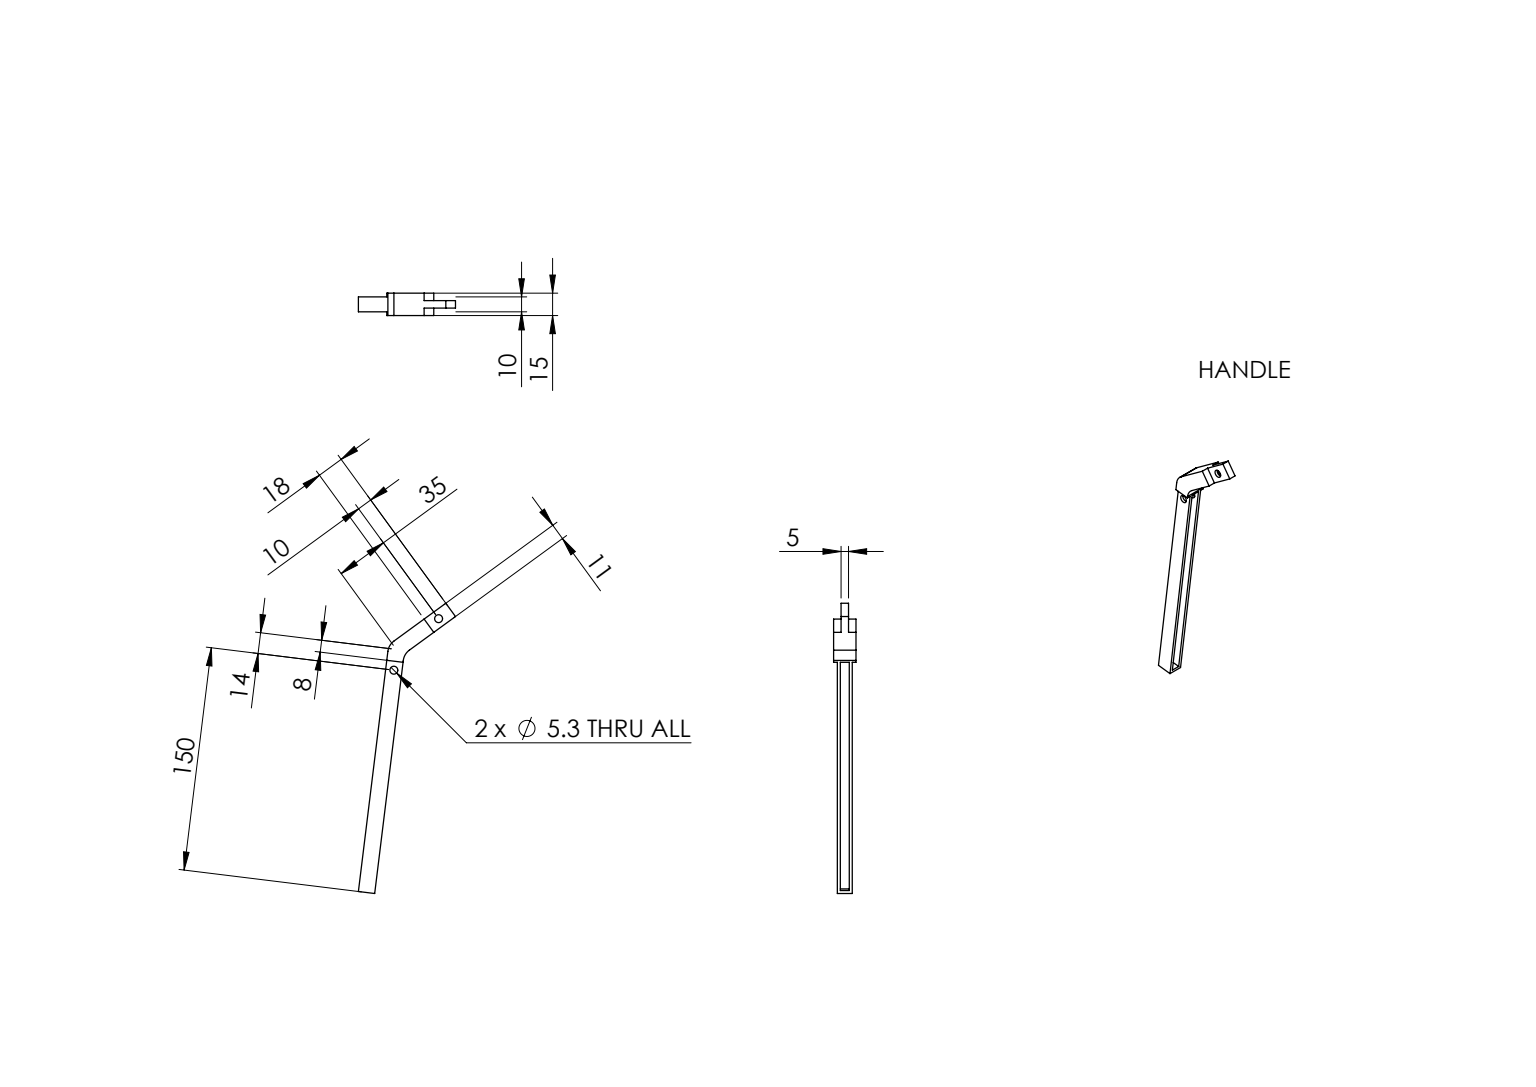
ISO-10303-21;
HEADER;
FILE_DESCRIPTION (('STEP AP214'),
    '1' );
FILE_NAME ('handle.step',
    '2026-10-31T03:36:27',
    ( '' ),
    ( '' ),
    'SwSTEP 2.0',
    'SolidWorks 2026',
    '' );
FILE_SCHEMA (( 'AUTOMOTIVE_DESIGN' ));
ENDSEC;

DATA;
#21=VERTEX_POINT ( 'NONE', #9252 ) ;
#62=EDGE_CURVE ( 'NONE', #31856, #6278, #12468, .T. ) ;
#113=VERTEX_POINT ( 'NONE', #15124 ) ;
#115=CARTESIAN_POINT ( 'NONE',  ( -98.52697526167152375, 63.53212182842481326, 3.000000000000000000 ) ) ;
#118=DIRECTION ( 'NONE',  ( -0.000000000000000000, 0.000000000000000000, 1.000000000000000000 ) ) ;
#138=PLANE ( 'NONE',  #16547 ) ;
#165=ADVANCED_FACE ( 'NONE', ( #28756 ), #138, .T. ) ;
#203=DIRECTION ( 'NONE',  ( 0.000000000000000000, 0.000000000000000000, -1.000000000000000000 ) ) ;
#232=ORIENTED_EDGE ( 'NONE', *, *, #9936, .F. ) ;
#254=ORIENTED_EDGE ( 'NONE', *, *, #1063, .F. ) ;
#301=LINE ( 'NONE', #23435, #5184 ) ;
#362=CYLINDRICAL_SURFACE ( 'NONE', #12150, 2.649999999999999467 ) ;
#375=FACE_OUTER_BOUND ( 'NONE', #36390, .T. ) ;
#384=FACE_BOUND ( 'NONE', #21248, .T. ) ;
#442=DIRECTION ( 'NONE',  ( 0.1219804832088915436, 0.9925324990730154395, 0.000000000000000000 ) ) ;
#456=VERTEX_POINT ( 'NONE', #12456 ) ;
#477=LINE ( 'NONE', #26256, #35797 ) ;
#513=DIRECTION ( 'NONE',  ( -0.8083506638593008775, -0.5887012860850803220, 0.000000000000000000 ) ) ;
#553=DIRECTION ( 'NONE',  ( 1.000000000000000000, 0.000000000000000000, 0.000000000000000000 ) ) ;
#622=EDGE_LOOP ( 'NONE', ( #9730, #27726, #18131, #5252 ) ) ;
#651=CARTESIAN_POINT ( 'NONE',  ( -70.80918835584510873, 215.2843023367891249, 3.000000000000000000 ) ) ;
#676=EDGE_CURVE ( 'NONE', #21562, #5473, #30076, .T. ) ;
#701=DIRECTION ( 'NONE',  ( 0.5887012860850814322, -0.8083506638592999893, 0.000000000000000000 ) ) ;
#743=DIRECTION ( 'NONE',  ( -0.000000000000000000, -0.000000000000000000, -1.000000000000000000 ) ) ;
#745=CARTESIAN_POINT ( 'NONE',  ( -44.35000000000001563, 244.5000000000000000, 5.000000000000000000 ) ) ;
#758=AXIS2_PLACEMENT_3D ( 'NONE', #36466, #33265, #18505 ) ;
#788=LINE ( 'NONE', #10083, #33967 ) ;
#790=EDGE_CURVE ( 'NONE', #30802, #1071, #21746, .T. ) ;
#796=LINE ( 'NONE', #12366, #13356 ) ;
#852=PLANE ( 'NONE',  #25668 ) ;
#858=AXIS2_PLACEMENT_3D ( 'NONE', #37408, #25218, #21126 ) ;
#894=EDGE_CURVE ( 'NONE', #12557, #11771, #34221, .T. ) ;
#916=AXIS2_PLACEMENT_3D ( 'NONE', #4687, #25159, #10753 ) ;
#946=CARTESIAN_POINT ( 'NONE',  ( -95.81998461310567450, 11.77610610744882358, 3.000000000000000000 ) ) ;
#1022=EDGE_CURVE ( 'NONE', #18726, #12845, #31747, .T. ) ;
#1057=LINE ( 'NONE', #12631, #35525 ) ;
#1063=EDGE_CURVE ( 'NONE', #6180, #9049, #14403, .T. ) ;
#1065=APPLICATION_CONTEXT ( 'automotive_design' ) ;
#1071=VERTEX_POINT ( 'NONE', #25874 ) ;
#1075=CARTESIAN_POINT ( 'NONE',  ( -76.95115755716804529, 229.4913094451872553, -7.500000000000000000 ) ) ;
#1204=AXIS2_PLACEMENT_3D ( 'NONE', #34736, #8411, #23189 ) ;
#1274=ORIENTED_EDGE ( 'NONE', *, *, #16176, .T. ) ;
#1330=ORIENTED_EDGE ( 'NONE', *, *, #23016, .T. ) ;
#1365=CARTESIAN_POINT ( 'NONE',  ( -89.83814373643217266, 60.44923248139874516, 5.000000000000000000 ) ) ;
#1475=VERTEX_POINT ( 'NONE', #13339 ) ;
#1483=VECTOR ( 'NONE', #7906, 1000.000000000000000 ) ;
#1499=LINE ( 'NONE', #745, #33419 ) ;
#1501=CARTESIAN_POINT ( 'NONE',  ( -60.72871937935236986, 215.3268752544371978, 5.000000000000000000 ) ) ;
#1550=DIRECTION ( 'NONE',  ( -0.9925324990730152175, 0.1219804832088933616, 0.000000000000000000 ) ) ;
#1568=ORIENTED_EDGE ( 'NONE', *, *, #4516, .F. ) ;
#1589=EDGE_CURVE ( 'NONE', #25013, #11771, #16193, .T. ) ;
#1594=DIRECTION ( 'NONE',  ( -1.558072081575740353E-16, -1.134704379232807653E-16, -1.000000000000000000 ) ) ;
#1616=DIRECTION ( 'NONE',  ( -0.000000000000000000, -0.000000000000000000, -1.000000000000000000 ) ) ;
#1652=FACE_OUTER_BOUND ( 'NONE', #9339, .T. ) ;
#1664=ORIENTED_EDGE ( 'NONE', *, *, #36317, .F. ) ;
#1688=LINE ( 'NONE', #24815, #8796 ) ;
#1716=CARTESIAN_POINT ( 'NONE',  ( -79.65000000000000568, 210.0000000000000000, 5.000000000000000888 ) ) ;
#1759=EDGE_CURVE ( 'NONE', #19165, #27793, #2654, .T. ) ;
#1782=DIRECTION ( 'NONE',  ( 1.000000000000000000, 0.000000000000000000, 0.000000000000000000 ) ) ;
#1788=ORIENTED_EDGE ( 'NONE', *, *, #3607, .F. ) ;
#1826=VECTOR ( 'NONE', #29654, 1000.000000000000114 ) ;
#1846=DIRECTION ( 'NONE',  ( -0.5887012860850813212, 0.8083506638592999893, 0.000000000000000000 ) ) ;
#1872=CARTESIAN_POINT ( 'NONE',  ( -74.35000000000002274, 210.0000000000000000, 3.000000000000000000 ) ) ;
#1885=DIRECTION ( 'NONE',  ( -0.000000000000000000, -0.000000000000000000, 1.000000000000000000 ) ) ;
#1893=DIRECTION ( 'NONE',  ( 1.000000000000000000, 0.000000000000000000, 0.000000000000000000 ) ) ;
#1965=CYLINDRICAL_SURFACE ( 'NONE', #29291, 2.649999999999992806 ) ;
#1966=CARTESIAN_POINT ( 'NONE',  ( -44.35000000000001563, 244.5000000000000000, -2.499999999999998224 ) ) ;
#1984=VERTEX_POINT ( 'NONE', #17641 ) ;
#2027=CARTESIAN_POINT ( 'NONE',  ( -74.35000000000002274, 210.0000000000000000, 5.000000000000000000 ) ) ;
#2063=ADVANCED_FACE ( 'NONE', ( #24072 ), #6442, .T. ) ;
#2067=ORIENTED_EDGE ( 'NONE', *, *, #6952, .T. ) ;
#2076=DIRECTION ( 'NONE',  ( 1.000000000000000000, 0.000000000000000000, 0.000000000000000000 ) ) ;
#2157=ORIENTED_EDGE ( 'NONE', *, *, #11690, .F. ) ;
#2200=PLANE ( 'NONE',  #31590 ) ;
#2202=DIRECTION ( 'NONE',  ( -1.000000000000000000, 0.000000000000000000, 0.000000000000000000 ) ) ;
#2225=ADVANCED_FACE ( 'NONE', ( #12877 ), #29745, .F. ) ;
#2246=DIRECTION ( 'NONE',  ( 0.000000000000000000, 0.000000000000000000, -1.000000000000000000 ) ) ;
#2286=DIRECTION ( 'NONE',  ( 0.000000000000000000, 0.000000000000000000, -1.000000000000000000 ) ) ;
#2390=CARTESIAN_POINT ( 'NONE',  ( -77.00000000000002842, 210.0000000000000000, -3.000000000000000000 ) ) ;
#2409=CARTESIAN_POINT ( 'NONE',  ( -82.45892874490161262, 210.6708926576488921, 5.000000000000000000 ) ) ;
#2412=EDGE_CURVE ( 'NONE', #21814, #23956, #15632, .T. ) ;
#2424=DIRECTION ( 'NONE',  ( -0.5887012860850800999, 0.8083506638593009885, 0.000000000000000000 ) ) ;
#2432=FACE_OUTER_BOUND ( 'NONE', #27389, .T. ) ;
#2469=CARTESIAN_POINT ( 'NONE',  ( -56.70466238434235606, 244.2363183625454894, -7.500000000000000000 ) ) ;
#2501=DIRECTION ( 'NONE',  ( 1.000000000000000000, 0.000000000000000000, 0.000000000000000000 ) ) ;
#2524=VECTOR ( 'NONE', #12034, 1000.000000000000000 ) ;
#2544=ORIENTED_EDGE ( 'NONE', *, *, #13634, .T. ) ;
#2564=ORIENTED_EDGE ( 'NONE', *, *, #9364, .F. ) ;
#2574=DIRECTION ( 'NONE',  ( -0.5887012860850800999, 0.8083506638593009885, -0.000000000000000000 ) ) ;
#2638=SHAPE_REPRESENTATION ( 'handle', ( #17215 ), #15973 ) ;
#2654=LINE ( 'NONE', #3216, #27316 ) ;
#2669=VECTOR ( 'NONE', #5948, 1000.000000000000000 ) ;
#2747=DIRECTION ( 'NONE',  ( -0.1219804832088935975, -0.9925324990730152175, 0.000000000000000000 ) ) ;
#2750=VECTOR ( 'NONE', #5758, 1000.000000000000000 ) ;
#2820=EDGE_LOOP ( 'NONE', ( #232, #22651, #21479, #3234 ) ) ;
#2857=ORIENTED_EDGE ( 'NONE', *, *, #34192, .F. ) ;
#2926=EDGE_CURVE ( 'NONE', #4785, #26168, #26714, .T. ) ;
#2932=DIRECTION ( 'NONE',  ( -1.000000000000000000, 0.000000000000000000, 1.636531581110199847E-16 ) ) ;
#2967=DIRECTION ( 'NONE',  ( -0.5887012860850802110, 0.8083506638593009885, 0.000000000000000000 ) ) ;
#2988=DIRECTION ( 'NONE',  ( -0.5887012860850802110, 0.8083506638593008775, 2.465190328815661618E-32 ) ) ;
#3046=ORIENTED_EDGE ( 'NONE', *, *, #24454, .T. ) ;
#3079=DIRECTION ( 'NONE',  ( -1.000000000000000000, 2.775557561562892929E-15, 0.000000000000000000 ) ) ;
#3082=PLANE ( 'NONE',  #1204 ) ;
#3099=ORIENTED_EDGE ( 'NONE', *, *, #7158, .T. ) ;
#3104=EDGE_CURVE ( 'NONE', #9049, #11398, #1499, .T. ) ;
#3106=DIRECTION ( 'NONE',  ( 0.1219804832088915436, 0.9925324990730154395, 0.000000000000000000 ) ) ;
#3138=AXIS2_PLACEMENT_3D ( 'NONE', #4717, #16110, #19522 ) ;
#3147=VERTEX_POINT ( 'NONE', #13825 ) ;
#3216=CARTESIAN_POINT ( 'NONE',  ( -74.35000000000002274, 210.0000000000000000, 5.000000000000000000 ) ) ;
#3234=ORIENTED_EDGE ( 'NONE', *, *, #32163, .F. ) ;
#3331=ORIENTED_EDGE ( 'NONE', *, *, #24454, .F. ) ;
#3343=ADVANCED_FACE ( 'NONE', ( #2432 ), #22730, .T. ) ;
#3349=EDGE_CURVE ( 'NONE', #18726, #12557, #28030, .T. ) ;
#3423=ORIENTED_EDGE ( 'NONE', *, *, #25829, .F. ) ;
#3598=CARTESIAN_POINT ( 'NONE',  ( -70.80918835584510873, 215.2843023367891249, 7.500000000000000000 ) ) ;
#3607=EDGE_CURVE ( 'NONE', #28581, #26637, #20070, .T. ) ;
#3645=LINE ( 'NONE', #6873, #19995 ) ;
#3688=CIRCLE ( 'NONE', #5491, 2.649999999999992806 ) ;
#3707=ORIENTED_EDGE ( 'NONE', *, *, #21878, .T. ) ;
#3805=AXIS2_PLACEMENT_3D ( 'NONE', #2409, #25905, #5616 ) ;
#3827=VERTEX_POINT ( 'NONE', #6976 ) ;
#3831=LINE ( 'NONE', #18826, #25418 ) ;
#3848=ORIENTED_EDGE ( 'NONE', *, *, #5518, .T. ) ;
#3850=ORIENTED_EDGE ( 'NONE', *, *, #8314, .T. ) ;
#3879=DIRECTION ( 'NONE',  ( -0.9925324990730152175, 0.1219804832088933616, 0.000000000000000000 ) ) ;
#3926=EDGE_CURVE ( 'NONE', #13097, #35545, #6587, .T. ) ;
#3932=DIRECTION ( 'NONE',  ( 0.9925324990730152175, -0.1219804832088933616, 0.000000000000000000 ) ) ;
#3950=AXIS2_PLACEMENT_3D ( 'NONE', #1501, #4347, #32971 ) ;
#3967=DIRECTION ( 'NONE',  ( -0.1219804832088933616, -0.9925324990730152175, 0.000000000000000000 ) ) ;
#3995=EDGE_LOOP ( 'NONE', ( #16459, #23432, #36012, #20738 ) ) ;
#3999=CIRCLE ( 'NONE', #28217, 2.649999999999999467 ) ;
#4055=ADVANCED_FACE ( 'NONE', ( #9806 ), #27055, .F. ) ;
#4063=VECTOR ( 'NONE', #21364, 1000.000000000000000 ) ;
#4074=ORIENTED_EDGE ( 'NONE', *, *, #23631, .F. ) ;
#4076=DIRECTION ( 'NONE',  ( -1.558072081575740353E-16, -1.134704379232807653E-16, -1.000000000000000000 ) ) ;
#4109=EDGE_LOOP ( 'NONE', ( #17978, #4758, #11450, #28178 ) ) ;
#4112=FACE_BOUND ( 'NONE', #26718, .T. ) ;
#4160=DIRECTION ( 'NONE',  ( -0.000000000000000000, -0.000000000000000000, 1.000000000000000000 ) ) ;
#4165=CARTESIAN_POINT ( 'NONE',  ( 25.01079625726091749, 203.5081962293401148, -5.000000000000000000 ) ) ;
#4229=CIRCLE ( 'NONE', #23608, 2.649999999999999467 ) ;
#4295=DIRECTION ( 'NONE',  ( 1.000000000000000000, 0.000000000000000000, 0.000000000000000000 ) ) ;
#4316=FACE_OUTER_BOUND ( 'NONE', #9865, .T. ) ;
#4344=DIRECTION ( 'NONE',  ( -0.9925324990730152175, 0.1219804832088933616, 0.000000000000000000 ) ) ;
#4347=DIRECTION ( 'NONE',  ( 0.000000000000000000, 0.000000000000000000, 1.000000000000000000 ) ) ;
#4367=ADVANCED_FACE ( 'NONE', ( #28170 ), #2200, .F. ) ;
#4393=PLANE ( 'NONE',  #29689 ) ;
#4397=CARTESIAN_POINT ( 'NONE',  ( -44.35000000000001563, 244.5000000000000000, 0.4999999999999995559 ) ) ;
#4410=ORIENTED_EDGE ( 'NONE', *, *, #6952, .F. ) ;
#4414=CIRCLE ( 'NONE', #34663, 2.649999999999999467 ) ;
#4423=CARTESIAN_POINT ( 'NONE',  ( -71.06414469631722852, 221.4078028065942476, -7.500000000000000888 ) ) ;
#4516=EDGE_CURVE ( 'NONE', #10660, #6278, #34966, .T. ) ;
#4546=CARTESIAN_POINT ( 'NONE',  ( -70.80918835584510873, 215.2843023367891249, -7.500000000000000000 ) ) ;
#4550=VERTEX_POINT ( 'NONE', #20205 ) ;
#4577=EDGE_CURVE ( 'NONE', #10335, #5564, #37064, .T. ) ;
#4625=LINE ( 'NONE', #9762, #14797 ) ;
#4643=DIRECTION ( 'NONE',  ( 0.000000000000000000, 0.000000000000000000, -1.000000000000000000 ) ) ;
#4651=DIRECTION ( 'NONE',  ( 0.000000000000000000, 0.000000000000000000, 1.000000000000000000 ) ) ;
#4661=ORIENTED_EDGE ( 'NONE', *, *, #25880, .F. ) ;
#4665=CARTESIAN_POINT ( 'NONE',  ( -70.80918835584510873, 215.2843023367891249, 7.500000000000000000 ) ) ;
#4681=VERTEX_POINT ( 'NONE', #22866 ) ;
#4687=CARTESIAN_POINT ( 'NONE',  ( -80.47386374675558329, 210.4269316912311183, 5.000000000000000000 ) ) ;
#4717=CARTESIAN_POINT ( 'NONE',  ( 38.04237167757703020, 114.1383727779938511, -2.499999999999996447 ) ) ;
#4722=VERTEX_POINT ( 'NONE', #29467 ) ;
#4736=ORIENTED_EDGE ( 'NONE', *, *, #8440, .F. ) ;
#4750=DIRECTION ( 'NONE',  ( -0.8083506638593009885, -0.5887012860850802110, 0.000000000000000000 ) ) ;
#4758=ORIENTED_EDGE ( 'NONE', *, *, #19169, .T. ) ;
#4785=VERTEX_POINT ( 'NONE', #651 ) ;
#4825=ORIENTED_EDGE ( 'NONE', *, *, #7158, .F. ) ;
#4865=DIRECTION ( 'NONE',  ( 1.000000000000000000, 0.000000000000000000, 0.000000000000000000 ) ) ;
#4942=EDGE_CURVE ( 'NONE', #14336, #33921, #9572, .T. ) ;
#5063=CIRCLE ( 'NONE', #33524, 9.999999999999994671 ) ;
#5102=CARTESIAN_POINT ( 'NONE',  ( -76.95115755716803108, 229.4913094451872553, 5.000000000000000000 ) ) ;
#5107=ORIENTED_EDGE ( 'NONE', *, *, #22482, .F. ) ;
#5134=ORIENTED_EDGE ( 'NONE', *, *, #8705, .F. ) ;
#5184=VECTOR ( 'NONE', #20982, 1000.000000000000000 ) ;
#5252=ORIENTED_EDGE ( 'NONE', *, *, #3926, .F. ) ;
#5262=EDGE_CURVE ( 'NONE', #21814, #456, #16018, .T. ) ;
#5314=FACE_OUTER_BOUND ( 'NONE', #26570, .T. ) ;
#5334=EDGE_LOOP ( 'NONE', ( #13000, #35007, #20837, #34063 ) ) ;
#5346=CARTESIAN_POINT ( 'NONE',  ( -47.00000000000000711, 244.5000000000000000, 5.000000000000000000 ) ) ;
#5348=CARTESIAN_POINT ( 'NONE',  ( -77.35272773637332477, 226.7246823105297153, -0.4999999999999908962 ) ) ;
#5426=EDGE_CURVE ( 'NONE', #1984, #18726, #26847, .T. ) ;
#5456=CARTESIAN_POINT ( 'NONE',  ( -50.22894823740646331, 235.3444610600932094, 7.500000000000000000 ) ) ;
#5473=VERTEX_POINT ( 'NONE', #34182 ) ;
#5491=AXIS2_PLACEMENT_3D ( 'NONE', #15956, #21462, #20892 ) ;
#5503=LINE ( 'NONE', #28625, #32722 ) ;
#5518=EDGE_CURVE ( 'NONE', #30233, #22653, #29035, .T. ) ;
#5524=CARTESIAN_POINT ( 'NONE',  ( -71.06414469631722852, 221.4078028065942476, 5.000000000000000000 ) ) ;
#5564=VERTEX_POINT ( 'NONE', #18257 ) ;
#5612=ORIENTED_EDGE ( 'NONE', *, *, #16982, .F. ) ;
#5616=DIRECTION ( 'NONE',  ( -0.1219804832088915297, -0.9925324990730154395, 0.000000000000000000 ) ) ;
#5758=DIRECTION ( 'NONE',  ( 0.000000000000000000, 0.000000000000000000, -1.000000000000000000 ) ) ;
#5889=ORIENTED_EDGE ( 'NONE', *, *, #4516, .T. ) ;
#5920=DIRECTION ( 'NONE',  ( -0.000000000000000000, -0.000000000000000000, -1.000000000000000000 ) ) ;
#5923=CARTESIAN_POINT ( 'NONE',  ( -44.35000000000001563, 244.5000000000000000, 2.500000000000000000 ) ) ;
#5948=DIRECTION ( 'NONE',  ( -0.000000000000000000, -0.000000000000000000, 1.000000000000000000 ) ) ;
#5989=ORIENTED_EDGE ( 'NONE', *, *, #7419, .T. ) ;
#6034=VERTEX_POINT ( 'NONE', #4397 ) ;
#6088=FACE_OUTER_BOUND ( 'NONE', #36886, .T. ) ;
#6146=VECTOR ( 'NONE', #20023, 1000.000000000000000 ) ;
#6168=ORIENTED_EDGE ( 'NONE', *, *, #36051, .F. ) ;
#6179=ORIENTED_EDGE ( 'NONE', *, *, #12556, .F. ) ;
#6180=VERTEX_POINT ( 'NONE', #31665 ) ;
#6181=LINE ( 'NONE', #11317, #36962 ) ;
#6217=DIRECTION ( 'NONE',  ( -1.000000000000000000, 0.000000000000000000, 0.000000000000000000 ) ) ;
#6261=ORIENTED_EDGE ( 'NONE', *, *, #32163, .T. ) ;
#6278=VERTEX_POINT ( 'NONE', #31481 ) ;
#6312=CARTESIAN_POINT ( 'NONE',  ( -71.54107125509844423, 209.3291073423510795, 5.000000000000000000 ) ) ;
#6342=ORIENTED_EDGE ( 'NONE', *, *, #1022, .T. ) ;
#6385=DIRECTION ( 'NONE',  ( -0.000000000000000000, -0.000000000000000000, 1.000000000000000000 ) ) ;
#6400=CARTESIAN_POINT ( 'NONE',  ( 50.97598229932587799, 123.5575933553551522, 0.5000000000000000000 ) ) ;
#6442=PLANE ( 'NONE',  #20666 ) ;
#6471=CARTESIAN_POINT ( 'NONE',  ( -104.7527771047627994, 12.87393045632884636, 3.000000000000000000 ) ) ;
#6587=LINE ( 'NONE', #6400, #30381 ) ;
#6592=LINE ( 'NONE', #10372, #19016 ) ;
#6712=EDGE_CURVE ( 'NONE', #4681, #15950, #10043, .T. ) ;
#6830=CARTESIAN_POINT ( 'NONE',  ( -100.7560012262353411, 61.79101779669657191, 5.000000000000000000 ) ) ;
#6833=EDGE_LOOP ( 'NONE', ( #5107, #6869, #12376, #22734 ) ) ;
#6834=ORIENTED_EDGE ( 'NONE', *, *, #25880, .T. ) ;
#6843=ORIENTED_EDGE ( 'NONE', *, *, #19169, .F. ) ;
#6869=ORIENTED_EDGE ( 'NONE', *, *, #4577, .T. ) ;
#6873=CARTESIAN_POINT ( 'NONE',  ( -73.23181873377778572, 221.0662276635146384, 0.4999999999999995559 ) ) ;
#6924=DIRECTION ( 'NONE',  ( -0.8083506638593009885, -0.5887012860850802110, 0.000000000000000000 ) ) ;
#6952=EDGE_CURVE ( 'NONE', #9049, #6180, #8223, .T. ) ;
#6970=PLANE ( 'NONE',  #36226 ) ;
#6976=CARTESIAN_POINT ( 'NONE',  ( -89.83814373643217266, 60.44923248139874516, 5.000000000000000000 ) ) ;
#6982=FACE_BOUND ( 'NONE', #30724, .T. ) ;
#7158=EDGE_CURVE ( 'NONE', #33921, #456, #25893, .T. ) ;
#7210=DIRECTION ( 'NONE',  ( 0.000000000000000000, 0.000000000000000000, -1.000000000000000000 ) ) ;
#7222=ORIENTED_EDGE ( 'NONE', *, *, #13634, .F. ) ;
#7229=ORIENTED_EDGE ( 'NONE', *, *, #25210, .T. ) ;
#7273=VECTOR ( 'NONE', #30741, 1000.000000000000000 ) ;
#7335=ADVANCED_FACE ( 'NONE', ( #35537, #20971 ), #852, .T. ) ;
#7337=CARTESIAN_POINT ( 'NONE',  ( -49.64999999999999858, 244.5000000000000000, 5.000000000000000000 ) ) ;
#7408=EDGE_CURVE ( 'NONE', #35545, #16460, #15649, .T. ) ;
#7419=EDGE_CURVE ( 'NONE', #456, #31856, #32884, .T. ) ;
#7436=ORIENTED_EDGE ( 'NONE', *, *, #7888, .F. ) ;
#7495=ORIENTED_EDGE ( 'NONE', *, *, #19453, .F. ) ;
#7524=DIRECTION ( 'NONE',  ( -0.1219804832088933616, -0.9925324990730152175, 0.000000000000000000 ) ) ;
#7542=ORIENTED_EDGE ( 'NONE', *, *, #17513, .F. ) ;
#7597=DIRECTION ( 'NONE',  ( -0.8083506638593009885, -0.5887012860850802110, 1.927470528863119295E-16 ) ) ;
#7606=AXIS2_PLACEMENT_3D ( 'NONE', #37260, #34791, #11308 ) ;
#7614=CARTESIAN_POINT ( 'NONE',  ( -50.22894823740646331, 235.3444610600932094, 5.000000000000000000 ) ) ;
#7652=DIRECTION ( 'NONE',  ( -1.000000000000000000, 0.000000000000000000, 0.000000000000000000 ) ) ;
#7734=ORIENTED_EDGE ( 'NONE', *, *, #37267, .F. ) ;
#7750=ADVANCED_FACE ( 'NONE', ( #11440 ), #14657, .T. ) ;
#7774=CARTESIAN_POINT ( 'NONE',  ( -77.00000000000002842, 210.0000000000000000, -5.000000000000001776 ) ) ;
#7785=AXIS2_PLACEMENT_3D ( 'NONE', #21330, #12780, #30219 ) ;
#7811=CARTESIAN_POINT ( 'NONE',  ( 38.04237167757703020, 114.1383727779938511, 0.5000000000000000000 ) ) ;
#7819=EDGE_LOOP ( 'NONE', ( #4410, #254 ) ) ;
#7866=CARTESIAN_POINT ( 'NONE',  ( -70.65404437008254490, 216.5466800865261234, 7.500000000000000000 ) ) ;
#7888=EDGE_CURVE ( 'NONE', #28581, #14336, #16520, .T. ) ;
#7906=DIRECTION ( 'NONE',  ( -0.1219804832088935975, -0.9925324990730152175, 0.000000000000000000 ) ) ;
#7915=VECTOR ( 'NONE', #20232, 1000.000000000000000 ) ;
#7926=FACE_OUTER_BOUND ( 'NONE', #9169, .T. ) ;
#7969=CARTESIAN_POINT ( 'NONE',  ( -42.15435043487494227, 254.8329415120769852, 5.000000000000000000 ) ) ;
#8017=DIRECTION ( 'NONE',  ( -0.8083506638593009885, -0.5887012860850802110, 1.927470528863119295E-16 ) ) ;
#8021=EDGE_LOOP ( 'NONE', ( #24673, #27021, #28004, #25561 ) ) ;
#8121=CARTESIAN_POINT ( 'NONE',  ( -50.22894823740646331, 235.3444610600932094, 7.500000000000000000 ) ) ;
#8141=DIRECTION ( 'NONE',  ( -0.8083506638593009885, -0.5887012860850802110, 1.927470528863119295E-16 ) ) ;
#8151=CARTESIAN_POINT ( 'NONE',  ( -89.59418277001439890, 62.43429747954478159, 5.000000000000000000 ) ) ;
#8156=CIRCLE ( 'NONE', #17840, 2.649999999999999467 ) ;
#8206=FILL_AREA_STYLE ('',( #14443 ) ) ;
#8223=CIRCLE ( 'NONE', #7606, 2.649999999999992806 ) ;
#8233=ORIENTED_EDGE ( 'NONE', *, *, #62, .T. ) ;
#8291=LINE ( 'NONE', #14712, #29370 ) ;
#8314=EDGE_CURVE ( 'NONE', #4722, #22653, #31026, .T. ) ;
#8362=DIRECTION ( 'NONE',  ( -0.9925324990730152175, 0.1219804832088933616, 0.000000000000000000 ) ) ;
#8366=ORIENTED_EDGE ( 'NONE', *, *, #26319, .F. ) ;
#8411=DIRECTION ( 'NONE',  ( -1.558072081575740353E-16, -1.134704379232807653E-16, -1.000000000000000000 ) ) ;
#8424=EDGE_CURVE ( 'NONE', #15950, #113, #8156, .T. ) ;
#8440=EDGE_CURVE ( 'NONE', #28968, #12845, #25513, .T. ) ;
#8446=CARTESIAN_POINT ( 'NONE',  ( -47.00000000000000711, 244.5000000000000000, -2.499999999999997780 ) ) ;
#8488=AXIS2_PLACEMENT_3D ( 'NONE', #19193, #24858, #36222 ) ;
#8496=CARTESIAN_POINT ( 'NONE',  ( -44.35000000000001563, 244.5000000000000000, -0.4999999999999982792 ) ) ;
#8519=ORIENTED_EDGE ( 'NONE', *, *, #20040, .F. ) ;
#8611=LINE ( 'NONE', #34014, #2750 ) ;
#8674=VECTOR ( 'NONE', #12592, 1000.000000000000000 ) ;
#8677=DIRECTION ( 'NONE',  ( 0.8083506638593009885, 0.5887012860850800999, 0.000000000000000000 ) ) ;
#8678=EDGE_CURVE ( 'NONE', #19208, #17150, #4625, .T. ) ;
#8705=EDGE_CURVE ( 'NONE', #37366, #17495, #9944, .T. ) ;
#8714=AXIS2_PLACEMENT_3D ( 'NONE', #16259, #30660, #4865 ) ;
#8776=CARTESIAN_POINT ( 'NONE',  ( -70.80918835584510873, 215.2843023367891249, 7.500000000000000000 ) ) ;
#8796=VECTOR ( 'NONE', #7210, 1000.000000000000000 ) ;
#8833=ORIENTED_EDGE ( 'NONE', *, *, #36051, .T. ) ;
#8890=ADVANCED_FACE ( 'NONE', ( #33071 ), #24169, .T. ) ;
#8945=( NAMED_UNIT ( * ) SI_UNIT ( $, .STERADIAN. ) SOLID_ANGLE_UNIT ( ) );
#9049=VERTEX_POINT ( 'NONE', #1966 ) ;
#9169=EDGE_LOOP ( 'NONE', ( #35167, #13770, #16487, #25746 ) ) ;
#9189=VERTEX_POINT ( 'NONE', #26390 ) ;
#9252=CARTESIAN_POINT ( 'NONE',  ( -79.65000000000001990, 210.0000000000000000, -5.000000000000001776 ) ) ;
#9289=DIRECTION ( 'NONE',  ( 0.9925324990730152175, -0.1219804832088933616, 0.000000000000000000 ) ) ;
#9334=VECTOR ( 'NONE', #701, 1000.000000000000114 ) ;
#9339=EDGE_LOOP ( 'NONE', ( #33249, #23101, #22001, #21854 ) ) ;
#9364=EDGE_CURVE ( 'NONE', #1475, #3147, #20916, .T. ) ;
#9444=DIRECTION ( 'NONE',  ( -0.1219804832088935975, -0.9925324990730152175, 0.000000000000000000 ) ) ;
#9495=ORIENTED_EDGE ( 'NONE', *, *, #20078, .F. ) ;
#9504=ORIENTED_EDGE ( 'NONE', *, *, #20322, .T. ) ;
#9562=VECTOR ( 'NONE', #2747, 1000.000000000000000 ) ;
#9572=LINE ( 'NONE', #35331, #2524 ) ;
#9574=ADVANCED_FACE ( 'NONE', ( #9726 ), #9904, .F. ) ;
#9582=DIRECTION ( 'NONE',  ( 0.000000000000000000, 0.000000000000000000, -1.000000000000000000 ) ) ;
#9626=FACE_OUTER_BOUND ( 'NONE', #24236, .T. ) ;
#9673=EDGE_CURVE ( 'NONE', #13899, #12159, #477, .T. ) ;
#9689=ORIENTED_EDGE ( 'NONE', *, *, #22347, .T. ) ;
#9703=ORIENTED_EDGE ( 'NONE', *, *, #21799, .F. ) ;
#9726=FACE_OUTER_BOUND ( 'NONE', #2820, .T. ) ;
#9729=DIRECTION ( 'NONE',  ( 0.9925324990730152175, -0.1219804832088933616, 0.000000000000000000 ) ) ;
#9730=ORIENTED_EDGE ( 'NONE', *, *, #19911, .F. ) ;
#9734=CARTESIAN_POINT ( 'NONE',  ( -81.72704584564829133, 216.6260876520869658, -5.000000000000000888 ) ) ;
#9762=CARTESIAN_POINT ( 'NONE',  ( 25.01079625726091749, 203.5081962293401148, 5.000000000000000000 ) ) ;
#9777=CARTESIAN_POINT ( 'NONE',  ( -55.52725981217221118, 242.6196170348268879, 0.4999999999999997780 ) ) ;
#9787=LINE ( 'NONE', #32903, #4063 ) ;
#9799=DIRECTION ( 'NONE',  ( -1.000000000000000000, 0.000000000000000000, -0.000000000000000000 ) ) ;
#9806=FACE_OUTER_BOUND ( 'NONE', #24174, .T. ) ;
#9823=ORIENTED_EDGE ( 'NONE', *, *, #35496, .T. ) ;
#9857=EDGE_CURVE ( 'NONE', #32744, #26637, #21377, .T. ) ;
#9859=DIRECTION ( 'NONE',  ( -0.000000000000000000, 0.000000000000000000, 1.000000000000000000 ) ) ;
#9865=EDGE_LOOP ( 'NONE', ( #7542, #36939, #8519, #10869 ) ) ;
#9897=DIRECTION ( 'NONE',  ( 0.8083506638593009885, 0.5887012860850802110, 0.000000000000000000 ) ) ;
#9904=CYLINDRICAL_SURFACE ( 'NONE', #20689, 2.649999999999992806 ) ;
#9907=ORIENTED_EDGE ( 'NONE', *, *, #37267, .T. ) ;
#9935=CARTESIAN_POINT ( 'NONE',  ( -80.98946968704737515, 222.6276076386831733, -7.500000000000000000 ) ) ;
#9936=EDGE_CURVE ( 'NONE', #30802, #6034, #21973, .T. ) ;
#9944=LINE ( 'NONE', #19057, #28021 ) ;
#10043=LINE ( 'NONE', #2027, #19125 ) ;
#10066=AXIS2_PLACEMENT_3D ( 'NONE', #31065, #16667, #10964 ) ;
#10083=CARTESIAN_POINT ( 'NONE',  ( -89.83814373643217266, 60.44923248139874516, 5.000000000000000000 ) ) ;
#10128=AXIS2_PLACEMENT_3D ( 'NONE', #5524, #28465, #20137 ) ;
#10222=DIRECTION ( 'NONE',  ( 0.000000000000000000, 0.000000000000000000, -1.000000000000000000 ) ) ;
#10226=DIRECTION ( 'NONE',  ( -0.9925324990730152175, 0.1219804832088933616, 0.000000000000000000 ) ) ;
#10238=ORIENTED_EDGE ( 'NONE', *, *, #23118, .F. ) ;
#10271=DIRECTION ( 'NONE',  ( -0.5887012860850814322, 0.8083506638593001004, 0.000000000000000000 ) ) ;
#10284=LINE ( 'NONE', #21495, #25755 ) ;
#10326=CARTESIAN_POINT ( 'NONE',  ( -42.59364919042334918, 252.0388376121882175, 0.5000000000000000000 ) ) ;
#10335=VERTEX_POINT ( 'NONE', #9777 ) ;
#10372=CARTESIAN_POINT ( 'NONE',  ( 25.01079625726091749, 203.5081962293401148, -3.000000000000000000 ) ) ;
#10384=ORIENTED_EDGE ( 'NONE', *, *, #3104, .T. ) ;
#10394=EDGE_CURVE ( 'NONE', #113, #15950, #4414, .T. ) ;
#10433=DIRECTION ( 'NONE',  ( 0.8083506638593009885, 0.5887012860850803220, -0.000000000000000000 ) ) ;
#10460=DIRECTION ( 'NONE',  ( 0.1219804832088915297, 0.9925324990730154395, 0.000000000000000000 ) ) ;
#10472=ORIENTED_EDGE ( 'NONE', *, *, #11690, .T. ) ;
#10482=CARTESIAN_POINT ( 'NONE',  ( -66.61573224020317241, 223.4103818930302054, 7.500000000000000000 ) ) ;
#10492=ORIENTED_EDGE ( 'NONE', *, *, #23719, .F. ) ;
#10513=ORIENTED_EDGE ( 'NONE', *, *, #29163, .T. ) ;
#10540=ORIENTED_EDGE ( 'NONE', *, *, #2412, .F. ) ;
#10544=CARTESIAN_POINT ( 'NONE',  ( -98.52697526167152375, 63.53212182842481326, -3.000000000000000000 ) ) ;
#10591=DIRECTION ( 'NONE',  ( 0.000000000000000000, 0.000000000000000000, -1.000000000000000000 ) ) ;
#10596=CARTESIAN_POINT ( 'NONE',  ( -49.64999999999999858, 244.5000000000000000, 0.4999999999999995559 ) ) ;
#10601=DIRECTION ( 'NONE',  ( 1.000000000000000000, 0.000000000000000000, 0.000000000000000000 ) ) ;
#10660=VERTEX_POINT ( 'NONE', #13032 ) ;
#10742=CARTESIAN_POINT ( 'NONE',  ( -42.15435043487492095, 254.8329415120769283, -2.500000000000000000 ) ) ;
#10753=DIRECTION ( 'NONE',  ( -0.1219804832088915297, -0.9925324990730154395, 0.000000000000000000 ) ) ;
#10796=LINE ( 'NONE', #27854, #27544 ) ;
#10808=CIRCLE ( 'NONE', #31983, 2.649999999999992806 ) ;
#10869=ORIENTED_EDGE ( 'NONE', *, *, #18419, .T. ) ;
#10889=ORIENTED_EDGE ( 'NONE', *, *, #62, .F. ) ;
#10918=VECTOR ( 'NONE', #35427, 1000.000000000000114 ) ;
#10928=DIRECTION ( 'NONE',  ( 0.000000000000000000, -0.000000000000000000, 1.000000000000000000 ) ) ;
#10946=CARTESIAN_POINT ( 'NONE',  ( -73.23181873377778572, 221.0662276635146384, 5.000000000000000000 ) ) ;
#10964=DIRECTION ( 'NONE',  ( -0.5887012860850802110, 0.8083506638593008775, 0.000000000000000000 ) ) ;
#11000=AXIS2_PLACEMENT_3D ( 'NONE', #21011, #15500, #29703 ) ;
#11079=EDGE_LOOP ( 'NONE', ( #11289, #14101 ) ) ;
#11082=CARTESIAN_POINT ( 'NONE',  ( -77.00000000000002842, 210.0000000000000000, -5.000000000000001776 ) ) ;
#11103=CARTESIAN_POINT ( 'NONE',  ( -80.75120197997713944, 224.5663476446710831, 7.500000000000000000 ) ) ;
#11150=VECTOR ( 'NONE', #3106, 1000.000000000000000 ) ;
#11155=LINE ( 'NONE', #11706, #30639 ) ;
#11193=AXIS2_PLACEMENT_3D ( 'NONE', #8151, #19533, #9729 ) ;
#11202=FACE_OUTER_BOUND ( 'NONE', #622, .T. ) ;
#11273=AXIS2_PLACEMENT_3D ( 'NONE', #4423, #27739, #7652 ) ;
#11283=VECTOR ( 'NONE', #24224, 1000.000000000000114 ) ;
#11289=ORIENTED_EDGE ( 'NONE', *, *, #25622, .T. ) ;
#11308=DIRECTION ( 'NONE',  ( -1.000000000000000000, 0.000000000000000000, 1.636531581110199847E-16 ) ) ;
#11317=CARTESIAN_POINT ( 'NONE',  ( 38.04237167757726468, 114.1383727779939647, -0.4999999999999965583 ) ) ;
#11377=DIRECTION ( 'NONE',  ( -1.000000000000000000, 0.000000000000000000, -0.000000000000000000 ) ) ;
#11398=VERTEX_POINT ( 'NONE', #8496 ) ;
#11440=FACE_OUTER_BOUND ( 'NONE', #29567, .T. ) ;
#11450=ORIENTED_EDGE ( 'NONE', *, *, #1759, .T. ) ;
#11618=ORIENTED_EDGE ( 'NONE', *, *, #25453, .T. ) ;
#11622=ORIENTED_EDGE ( 'NONE', *, *, #30740, .F. ) ;
#11667=ORIENTED_EDGE ( 'NONE', *, *, #9857, .F. ) ;
#11686=LINE ( 'NONE', #23439, #7915 ) ;
#11690=EDGE_CURVE ( 'NONE', #14163, #1071, #25954, .T. ) ;
#11695=CARTESIAN_POINT ( 'NONE',  ( 52.59268362704444399, 124.7349959275252615, -2.500000000000000000 ) ) ;
#11706=CARTESIAN_POINT ( 'NONE',  ( -43.77105176259354380, 253.6555389399068190, -0.4999999999999995559 ) ) ;
#11771=VERTEX_POINT ( 'NONE', #30464 ) ;
#11795=EDGE_LOOP ( 'NONE', ( #35466, #7229, #18055, #35121 ) ) ;
#11818=VERTEX_POINT ( 'NONE', #1075 ) ;
#11857=DIRECTION ( 'NONE',  ( -0.9925324990730152175, 0.1219804832088933616, 0.000000000000000000 ) ) ;
#11878=ADVANCED_FACE ( 'NONE', ( #24209, #4112 ), #6970, .T. ) ;
#12005=VERTEX_POINT ( 'NONE', #27979 ) ;
#12034=DIRECTION ( 'NONE',  ( -0.5887012860850800999, 0.8083506638593009885, -0.000000000000000000 ) ) ;
#12081=CARTESIAN_POINT ( 'NONE',  ( -89.59418277001438469, 62.43429747954478159, 3.000000000000000000 ) ) ;
#12086=CARTESIAN_POINT ( 'NONE',  ( -77.00000000000002842, 210.0000000000000000, 3.000000000000000000 ) ) ;
#12134=ADVANCED_FACE ( 'NONE', ( #37059 ), #25322, .T. ) ;
#12150=AXIS2_PLACEMENT_3D ( 'NONE', #23312, #20476, #29164 ) ;
#12159=VERTEX_POINT ( 'NONE', #10544 ) ;
#12182=ORIENTED_EDGE ( 'NONE', *, *, #33078, .F. ) ;
#12192=ORIENTED_EDGE ( 'NONE', *, *, #1022, .F. ) ;
#12316=DIRECTION ( 'NONE',  ( -0.000000000000000000, -0.000000000000000000, 1.000000000000000000 ) ) ;
#12336=AXIS2_PLACEMENT_3D ( 'NONE', #12467, #21389, #3932 ) ;
#12347=CARTESIAN_POINT ( 'NONE',  ( -42.59364919042334918, 252.0388376121882175, -0.4999999999999995559 ) ) ;
#12366=CARTESIAN_POINT ( 'NONE',  ( -81.72704584564829133, 216.6260876520869658, 7.500000000000000000 ) ) ;
#12376=ORIENTED_EDGE ( 'NONE', *, *, #16176, .F. ) ;
#12411=CIRCLE ( 'NONE', #19179, 2.649999999999999467 ) ;
#12456=CARTESIAN_POINT ( 'NONE',  ( -42.15435043487492095, 254.8329415120769283, 2.500000000000000000 ) ) ;
#12467=CARTESIAN_POINT ( 'NONE',  ( -70.80918835584510873, 215.2843023367891249, 7.500000000000000000 ) ) ;
#12468=LINE ( 'NONE', #29522, #28029 ) ;
#12501=VECTOR ( 'NONE', #32459, 1000.000000000000114 ) ;
#12536=VECTOR ( 'NONE', #18296, 1000.000000000000000 ) ;
#12556=EDGE_CURVE ( 'NONE', #33064, #27793, #31365, .T. ) ;
#12557=VERTEX_POINT ( 'NONE', #9935 ) ;
#12576=ORIENTED_EDGE ( 'NONE', *, *, #5426, .T. ) ;
#12592=DIRECTION ( 'NONE',  ( -0.000000000000000000, -0.000000000000000000, -1.000000000000000000 ) ) ;
#12631=CARTESIAN_POINT ( 'NONE',  ( -50.22894823740646331, 235.3444610600932094, 5.000000000000000000 ) ) ;
#12659=CARTESIAN_POINT ( 'NONE',  ( -56.70466238434235606, 244.2363183625454894, 7.500000000000000000 ) ) ;
#12702=DIRECTION ( 'NONE',  ( 1.000000000000000000, 0.000000000000000000, 0.000000000000000000 ) ) ;
#12718=ORIENTED_EDGE ( 'NONE', *, *, #20728, .T. ) ;
#12743=ORIENTED_EDGE ( 'NONE', *, *, #894, .T. ) ;
#12780=DIRECTION ( 'NONE',  ( -0.000000000000000000, -0.000000000000000000, 1.000000000000000000 ) ) ;
#12795=CARTESIAN_POINT ( 'NONE',  ( -42.15435043487494227, 254.8329415120769852, 5.000000000000000000 ) ) ;
#12800=ORIENTED_EDGE ( 'NONE', *, *, #19147, .F. ) ;
#12821=CYLINDRICAL_SURFACE ( 'NONE', #31848, 2.649999999999999467 ) ;
#12841=DIRECTION ( 'NONE',  ( -1.000000000000000000, 0.000000000000000000, -0.000000000000000000 ) ) ;
#12845=VERTEX_POINT ( 'NONE', #15450 ) ;
#12856=ORIENTED_EDGE ( 'NONE', *, *, #3607, .T. ) ;
#12859=EDGE_CURVE ( 'NONE', #19808, #11398, #10808, .T. ) ;
#12877=FACE_OUTER_BOUND ( 'NONE', #4109, .T. ) ;
#12901=ORIENTED_EDGE ( 'NONE', *, *, #10394, .T. ) ;
#13000=ORIENTED_EDGE ( 'NONE', *, *, #25210, .F. ) ;
#13032=CARTESIAN_POINT ( 'NONE',  ( -50.22894823740647752, 235.3444610600932094, -2.499999999999996447 ) ) ;
#13046=FACE_OUTER_BOUND ( 'NONE', #17684, .T. ) ;
#13097=VERTEX_POINT ( 'NONE', #14058 ) ;
#13145=( NAMED_UNIT ( * ) PLANE_ANGLE_UNIT ( ) SI_UNIT ( $, .RADIAN. ) );
#13271=DIRECTION ( 'NONE',  ( -0.000000000000000000, -0.000000000000000000, 1.000000000000000000 ) ) ;
#13275=ORIENTED_EDGE ( 'NONE', *, *, #36317, .T. ) ;
#13299=LINE ( 'NONE', #31291, #7273 ) ;
#13339=CARTESIAN_POINT ( 'NONE',  ( -50.22894823740646331, 235.3444610600932094, -7.500000000000000000 ) ) ;
#13350=FACE_OUTER_BOUND ( 'NONE', #33443, .T. ) ;
#13356=VECTOR ( 'NONE', #27149, 1000.000000000000000 ) ;
#13487=CARTESIAN_POINT ( 'NONE',  ( -89.83814373643217266, 60.44923248139874516, -5.000000000000000000 ) ) ;
#13580=DIRECTION ( 'NONE',  ( -0.9925324990730152175, 0.1219804832088933616, 0.000000000000000000 ) ) ;
#13634=EDGE_CURVE ( 'NONE', #15181, #17150, #37022, .T. ) ;
#13650=VECTOR ( 'NONE', #8141, 1000.000000000000114 ) ;
#13668=DIRECTION ( 'NONE',  ( -0.5887012860850802110, 0.8083506638593009885, 0.000000000000000000 ) ) ;
#13672=VECTOR ( 'NONE', #34605, 1000.000000000000000 ) ;
#13678=VECTOR ( 'NONE', #1616, 1000.000000000000000 ) ;
#13709=FACE_OUTER_BOUND ( 'NONE', #15135, .T. ) ;
#13770=ORIENTED_EDGE ( 'NONE', *, *, #19911, .T. ) ;
#13780=DIRECTION ( 'NONE',  ( -1.000000000000000000, 0.000000000000000000, 0.000000000000000000 ) ) ;
#13823=DIRECTION ( 'NONE',  ( -1.000000000000000000, 0.000000000000000000, 0.000000000000000000 ) ) ;
#13825=CARTESIAN_POINT ( 'NONE',  ( -66.61573224020317241, 223.4103818930302054, -7.500000000000000000 ) ) ;
#13831=CIRCLE ( 'NONE', #34994, 2.649999999999992806 ) ;
#13895=( LENGTH_UNIT ( ) NAMED_UNIT ( * ) SI_UNIT ( .MILLI., .METRE. ) );
#13899=VERTEX_POINT ( 'NONE', #35655 ) ;
#13914=DIRECTION ( 'NONE',  ( -0.000000000000000000, -0.000000000000000000, 1.000000000000000000 ) ) ;
#13921=ORIENTED_EDGE ( 'NONE', *, *, #7419, .F. ) ;
#13967=FACE_OUTER_BOUND ( 'NONE', #16034, .T. ) ;
#14023=ORIENTED_EDGE ( 'NONE', *, *, #23631, .T. ) ;
#14048=LINE ( 'NONE', #22768, #33301 ) ;
#14058=CARTESIAN_POINT ( 'NONE',  ( -38.47274018782781013, 246.3803829651731121, 0.5000000000000000000 ) ) ;
#14064=ORIENTED_EDGE ( 'NONE', *, *, #1589, .T. ) ;
#14076=LINE ( 'NONE', #5348, #23030 ) ;
#14095=CARTESIAN_POINT ( 'NONE',  ( -47.00000000000000711, 244.5000000000000000, 5.000000000000000000 ) ) ;
#14101=ORIENTED_EDGE ( 'NONE', *, *, #22629, .T. ) ;
#14112=ORIENTED_EDGE ( 'NONE', *, *, #2926, .T. ) ;
#14129=ADVANCED_FACE ( 'NONE', ( #20351, #31708 ), #3082, .F. ) ;
#14160=AXIS2_PLACEMENT_3D ( 'NONE', #21203, #24221, #12841 ) ;
#14163=VERTEX_POINT ( 'NONE', #5923 ) ;
#14230=DIRECTION ( 'NONE',  ( -0.000000000000000000, -0.000000000000000000, 1.000000000000000000 ) ) ;
#14236=ORIENTED_EDGE ( 'NONE', *, *, #1063, .T. ) ;
#14291=ORIENTED_EDGE ( 'NONE', *, *, #8678, .T. ) ;
#14314=AXIS2_PLACEMENT_3D ( 'NONE', #6312, #29429, #34925 ) ;
#14336=VERTEX_POINT ( 'NONE', #18455 ) ;
#14397=PRODUCT_DEFINITION_SHAPE ( 'NONE', 'NONE',  #18078 ) ;
#14403=CIRCLE ( 'NONE', #32553, 2.649999999999992806 ) ;
#14404=LINE ( 'NONE', #30531, #27287 ) ;
#14443=FILL_AREA_STYLE_COLOUR ( '', #15373 ) ;
#14545=( GEOMETRIC_REPRESENTATION_CONTEXT ( 3 ) GLOBAL_UNCERTAINTY_ASSIGNED_CONTEXT ( ( #16549 ) ) GLOBAL_UNIT_ASSIGNED_CONTEXT ( ( #24444, #24992, #36549 ) ) REPRESENTATION_CONTEXT ( 'NONE', 'WORKASPACE' ) );
#14615=CARTESIAN_POINT ( 'NONE',  ( 0.000000000000000000, 0.000000000000000000, -7.500000000000000000 ) ) ;
#14634=EDGE_LOOP ( 'NONE', ( #28158, #32281, #13921, #23905 ) ) ;
#14657=PLANE ( 'NONE',  #17212 ) ;
#14712=CARTESIAN_POINT ( 'NONE',  ( -71.54107125509844423, 209.3291073423510795, 5.000000000000000000 ) ) ;
#14797=VECTOR ( 'NONE', #24720, 1000.000000000000114 ) ;
#14807=FACE_OUTER_BOUND ( 'NONE', #19683, .T. ) ;
#14824=DIRECTION ( 'NONE',  ( -1.000000000000000000, 0.000000000000000000, -0.000000000000000000 ) ) ;
#14865=CARTESIAN_POINT ( 'NONE',  ( -71.54107125509844423, 209.3291073423510795, -5.000000000000000000 ) ) ;
#14879=CIRCLE ( 'NONE', #34843, 2.649999999999999467 ) ;
#15023=CARTESIAN_POINT ( 'NONE',  ( -49.64999999999999858, 244.5000000000000000, -0.4999999999999973910 ) ) ;
#15033=CARTESIAN_POINT ( 'NONE',  ( -95.81998461310567450, 11.77610610744882358, -3.000000000000000000 ) ) ;
#15124=CARTESIAN_POINT ( 'NONE',  ( -79.65000000000001990, 210.0000000000000000, -3.000000000000000000 ) ) ;
#15135=EDGE_LOOP ( 'NONE', ( #2067, #9504, #28736, #24048 ) ) ;
#15181=VERTEX_POINT ( 'NONE', #6830 ) ;
#15269=CARTESIAN_POINT ( 'NONE',  ( 52.59268362704444399, 124.7349959275252615, -2.500000000000000000 ) ) ;
#15295=PRODUCT_CONTEXT ( 'NONE', #1065, 'mechanical' ) ;
#15373=COLOUR_RGB ( '',0.8941176470588234615, 0.8941176470588234615, 0.8941176470588234615 ) ;
#15429=EDGE_CURVE ( 'NONE', #13097, #33922, #11686, .T. ) ;
#15450=CARTESIAN_POINT ( 'NONE',  ( -81.72704584564829133, 216.6260876520869658, 7.500000000000000000 ) ) ;
#15454=VECTOR ( 'NONE', #18932, 1000.000000000000000 ) ;
#15493=DIRECTION ( 'NONE',  ( -0.000000000000000000, 0.000000000000000000, 1.000000000000000000 ) ) ;
#15500=DIRECTION ( 'NONE',  ( -0.000000000000000000, -0.000000000000000000, 1.000000000000000000 ) ) ;
#15517=ADVANCED_FACE ( 'NONE', ( #26458 ), #28931, .F. ) ;
#15551=AXIS2_PLACEMENT_3D ( 'NONE', #20103, #16708, #11377 ) ;
#15632=LINE ( 'NONE', #18109, #12536 ) ;
#15649=LINE ( 'NONE', #27197, #27490 ) ;
#15661=DIRECTION ( 'NONE',  ( -1.000000000000000000, 0.000000000000000000, 0.000000000000000000 ) ) ;
#15683=CARTESIAN_POINT ( 'NONE',  ( -89.83814373643217266, 60.44923248139874516, -5.000000000000000000 ) ) ;
#15733=CARTESIAN_POINT ( 'NONE',  ( 25.01079625726091749, 203.5081962293401148, 3.000000000000000000 ) ) ;
#15866=FACE_OUTER_BOUND ( 'NONE', #11795, .T. ) ;
#15870=ORIENTED_EDGE ( 'NONE', *, *, #31837, .F. ) ;
#15872=CARTESIAN_POINT ( 'NONE',  ( -47.00000000000000711, 244.5000000000000000, 2.500000000000000000 ) ) ;
#15899=EDGE_LOOP ( 'NONE', ( #35215, #18022 ) ) ;
#15950=VERTEX_POINT ( 'NONE', #25067 ) ;
#15956=CARTESIAN_POINT ( 'NONE',  ( -47.00000000000000711, 244.5000000000000000, -0.4999999999999978351 ) ) ;
#15973=( GEOMETRIC_REPRESENTATION_CONTEXT ( 3 ) GLOBAL_UNCERTAINTY_ASSIGNED_CONTEXT ( ( #21478 ) ) GLOBAL_UNIT_ASSIGNED_CONTEXT ( ( #33793, #13145, #22054 ) ) REPRESENTATION_CONTEXT ( 'NONE', 'WORKASPACE' ) );
#16018=LINE ( 'NONE', #22446, #17174 ) ;
#16021=CARTESIAN_POINT ( 'NONE',  ( -44.35000000000001563, 244.5000000000000000, 5.000000000000000000 ) ) ;
#16034=EDGE_LOOP ( 'NONE', ( #32366, #6168, #6261, #10472 ) ) ;
#16047=CARTESIAN_POINT ( 'NONE',  ( 0.000000000000000000, 0.000000000000000000, 0.000000000000000000 ) ) ;
#16068=DIRECTION ( 'NONE',  ( 0.000000000000000000, 0.000000000000000000, -1.000000000000000000 ) ) ;
#16108=LINE ( 'NONE', #27841, #18186 ) ;
#16110=DIRECTION ( 'NONE',  ( 0.8083506638593009885, 0.5887012860850800999, 0.000000000000000000 ) ) ;
#16176=EDGE_CURVE ( 'NONE', #16460, #5564, #14076, .T. ) ;
#16193=LINE ( 'NONE', #27743, #8674 ) ;
#16222=CARTESIAN_POINT ( 'NONE',  ( -77.00000000000002842, 210.0000000000000000, -3.000000000000000000 ) ) ;
#16233=VECTOR ( 'NONE', #30462, 1000.000000000000000 ) ;
#16259=CARTESIAN_POINT ( 'NONE',  ( -47.00000000000000711, 244.5000000000000000, 5.000000000000000000 ) ) ;
#16307=FACE_OUTER_BOUND ( 'NONE', #25109, .T. ) ;
#16347=CARTESIAN_POINT ( 'NONE',  ( -56.70466238434234185, 244.2363183625454894, 2.500000000000000000 ) ) ;
#16362=ADVANCED_FACE ( 'NONE', ( #32059, #6088 ), #17672, .F. ) ;
#16456=EDGE_CURVE ( 'NONE', #11398, #19808, #3688, .T. ) ;
#16459=ORIENTED_EDGE ( 'NONE', *, *, #15429, .F. ) ;
#16460=VERTEX_POINT ( 'NONE', #12347 ) ;
#16487=ORIENTED_EDGE ( 'NONE', *, *, #15429, .T. ) ;
#16520=LINE ( 'NONE', #7614, #16597 ) ;
#16547=AXIS2_PLACEMENT_3D ( 'NONE', #22533, #8677, #2424 ) ;
#16549=UNCERTAINTY_MEASURE_WITH_UNIT (LENGTH_MEASURE( 1.000000000000000082E-05 ), #24444, 'distance_accuracy_value', 'NONE');
#16597=VECTOR ( 'NONE', #2286, 1000.000000000000000 ) ;
#16598=DIRECTION ( 'NONE',  ( -0.000000000000000000, -0.000000000000000000, 1.000000000000000000 ) ) ;
#16630=DIRECTION ( 'NONE',  ( 0.000000000000000000, 0.000000000000000000, -1.000000000000000000 ) ) ;
#16667=DIRECTION ( 'NONE',  ( 0.8083506638593009885, 0.5887012860850803220, -0.000000000000000000 ) ) ;
#16670=CARTESIAN_POINT ( 'NONE',  ( -80.98946968704737515, 222.6276076386831733, 5.000000000000000000 ) ) ;
#16708=DIRECTION ( 'NONE',  ( 0.000000000000000000, 0.000000000000000000, -1.000000000000000000 ) ) ;
#16797=VECTOR ( 'NONE', #7597, 1000.000000000000114 ) ;
#16879=LINE ( 'NONE', #19735, #16797 ) ;
#16924=DIRECTION ( 'NONE',  ( -0.000000000000000000, -0.000000000000000000, 1.000000000000000000 ) ) ;
#16982=EDGE_CURVE ( 'NONE', #6278, #27573, #14404, .T. ) ;
#16986=AXIS2_PLACEMENT_3D ( 'NONE', #14615, #203, #34515 ) ;
#17040=CARTESIAN_POINT ( 'NONE',  ( -73.23181873377778572, 221.0662276635146384, -0.4999999999999908962 ) ) ;
#17043=AXIS2_PLACEMENT_3D ( 'NONE', #30128, #4160, #553 ) ;
#17078=ADVANCED_FACE ( 'NONE', ( #26326 ), #362, .F. ) ;
#17087=VECTOR ( 'NONE', #513, 1000.000000000000114 ) ;
#17150=VERTEX_POINT ( 'NONE', #21042 ) ;
#17174=VECTOR ( 'NONE', #33993, 1000.000000000000000 ) ;
#17212=AXIS2_PLACEMENT_3D ( 'NONE', #26208, #31715, #25472 ) ;
#17215=AXIS2_PLACEMENT_3D ( 'NONE', #16047, #4651, #19645 ) ;
#17219=CIRCLE ( 'NONE', #858, 2.649999999999992806 ) ;
#17269=CARTESIAN_POINT ( 'NONE',  ( -79.74198084750221938, 216.3821266856691921, 3.000000000000000000 ) ) ;
#17338=VECTOR ( 'NONE', #23268, 1000.000000000000000 ) ;
#17495=VERTEX_POINT ( 'NONE', #115 ) ;
#17513=EDGE_CURVE ( 'NONE', #5564, #22630, #6181, .T. ) ;
#17575=VECTOR ( 'NONE', #22642, 1000.000000000000000 ) ;
#17641=CARTESIAN_POINT ( 'NONE',  ( -76.95115755716804529, 229.4913094451872553, 7.500000000000000000 ) ) ;
#17672=PLANE ( 'NONE',  #20050 ) ;
#17684=EDGE_LOOP ( 'NONE', ( #37031, #13275, #27813, #14023 ) ) ;
#17707=CARTESIAN_POINT ( 'NONE',  ( -56.70466238434235606, 244.2363183625454894, 7.500000000000000000 ) ) ;
#17712=LINE ( 'NONE', #20377, #2669 ) ;
#17840=AXIS2_PLACEMENT_3D ( 'NONE', #2390, #16630, #2202 ) ;
#17978=ORIENTED_EDGE ( 'NONE', *, *, #29163, .F. ) ;
#18022=ORIENTED_EDGE ( 'NONE', *, *, #12859, .T. ) ;
#18055=ORIENTED_EDGE ( 'NONE', *, *, #8424, .F. ) ;
#18078=PRODUCT_DEFINITION ( 'UNKNOWN', '', #19036, #21021 ) ;
#18089=LINE ( 'NONE', #20740, #28195 ) ;
#18109=CARTESIAN_POINT ( 'NONE',  ( -35.67863628793905661, 245.9410842096246483, 5.000000000000000000 ) ) ;
#18128=EDGE_CURVE ( 'NONE', #3827, #21562, #788, .T. ) ;
#18131=ORIENTED_EDGE ( 'NONE', *, *, #22482, .T. ) ;
#18186=VECTOR ( 'NONE', #10222, 1000.000000000000000 ) ;
#18211=VECTOR ( 'NONE', #10271, 999.9999999999998863 ) ;
#18218=LINE ( 'NONE', #946, #26338 ) ;
#18257=CARTESIAN_POINT ( 'NONE',  ( -55.52725981217218276, 242.6196170348268879, -0.4999999999999978351 ) ) ;
#18296=DIRECTION ( 'NONE',  ( -0.000000000000000000, -0.000000000000000000, -1.000000000000000000 ) ) ;
#18303=DIRECTION ( 'NONE',  ( -0.5887012860850802110, 0.8083506638593009885, 0.000000000000000000 ) ) ;
#18390=CARTESIAN_POINT ( 'NONE',  ( -89.83814373643217266, 60.44923248139874516, 5.000000000000000000 ) ) ;
#18405=EDGE_CURVE ( 'NONE', #27793, #33064, #36314, .T. ) ;
#18419=EDGE_CURVE ( 'NONE', #4550, #22630, #13299, .T. ) ;
#18455=CARTESIAN_POINT ( 'NONE',  ( -50.22894823740647041, 235.3444610600932094, 2.500000000000000000 ) ) ;
#18498=LINE ( 'NONE', #16021, #22626 ) ;
#18505=DIRECTION ( 'NONE',  ( -1.000000000000000000, 0.000000000000000000, 0.000000000000000000 ) ) ;
#18623=AXIS2_PLACEMENT_3D ( 'NONE', #7969, #10433, #19361 ) ;
#18649=ORIENTED_EDGE ( 'NONE', *, *, #894, .F. ) ;
#18726=VERTEX_POINT ( 'NONE', #20669 ) ;
#18763=EDGE_CURVE ( 'NONE', #22653, #11771, #14048, .T. ) ;
#18794=VECTOR ( 'NONE', #743, 1000.000000000000000 ) ;
#18826=CARTESIAN_POINT ( 'NONE',  ( -56.70466238434235606, 244.2363183625454894, 7.500000000000000000 ) ) ;
#18871=DIRECTION ( 'NONE',  ( -0.000000000000000000, -0.000000000000000000, 1.000000000000000000 ) ) ;
#18932=DIRECTION ( 'NONE',  ( -0.000000000000000000, -0.000000000000000000, -1.000000000000000000 ) ) ;
#18964=ORIENTED_EDGE ( 'NONE', *, *, #21799, .T. ) ;
#19016=VECTOR ( 'NONE', #21576, 1000.000000000000114 ) ;
#19026=EDGE_CURVE ( 'NONE', #28968, #19208, #24073, .T. ) ;
#19036=PRODUCT_DEFINITION_FORMATION_WITH_SPECIFIED_SOURCE ( 'ANY', '', #28294, .NOT_KNOWN. ) ;
#19057=CARTESIAN_POINT ( 'NONE',  ( 6.225801843091343102, 50.65819137209577150, 3.000000000000000000 ) ) ;
#19099=DIRECTION ( 'NONE',  ( 0.9925324990730152175, -0.1219804832088933616, 0.000000000000000000 ) ) ;
#19125=VECTOR ( 'NONE', #21620, 1000.000000000000000 ) ;
#19147=EDGE_CURVE ( 'NONE', #37366, #13899, #16108, .T. ) ;
#19154=ORIENTED_EDGE ( 'NONE', *, *, #24982, .T. ) ;
#19165=VERTEX_POINT ( 'NONE', #1872 ) ;
#19169=EDGE_CURVE ( 'NONE', #9189, #19165, #4229, .T. ) ;
#19178=PLANE ( 'NONE',  #25676 ) ;
#19179=AXIS2_PLACEMENT_3D ( 'NONE', #7774, #13271, #2076 ) ;
#19193=CARTESIAN_POINT ( 'NONE',  ( -77.00000000000002842, 210.0000000000000000, 5.000000000000000888 ) ) ;
#19208=VERTEX_POINT ( 'NONE', #19338 ) ;
#19230=CARTESIAN_POINT ( 'NONE',  ( -70.80918835584510873, 215.2843023367891249, -5.000000000000000888 ) ) ;
#19264=ORIENTED_EDGE ( 'NONE', *, *, #3349, .F. ) ;
#19313=LINE ( 'NONE', #30851, #15454 ) ;
#19338=CARTESIAN_POINT ( 'NONE',  ( -70.80918835584509452, 215.2843023367891249, 5.000000000000000000 ) ) ;
#19361=DIRECTION ( 'NONE',  ( -0.5887012860850802110, 0.8083506638593008775, 0.000000000000000000 ) ) ;
#19453=EDGE_CURVE ( 'NONE', #27573, #11818, #23600, .T. ) ;
#19512=VECTOR ( 'NONE', #4344, 1000.000000000000114 ) ;
#19522=DIRECTION ( 'NONE',  ( -0.5887012860850800999, 0.8083506638593009885, 0.000000000000000000 ) ) ;
#19533=DIRECTION ( 'NONE',  ( -0.1219804832088933616, -0.9925324990730152175, 0.000000000000000000 ) ) ;
#19584=ORIENTED_EDGE ( 'NONE', *, *, #12859, .F. ) ;
#19607=ORIENTED_EDGE ( 'NONE', *, *, #20933, .T. ) ;
#19645=DIRECTION ( 'NONE',  ( 1.000000000000000000, 0.000000000000000000, 0.000000000000000000 ) ) ;
#19683=EDGE_LOOP ( 'NONE', ( #18649, #26215, #7495, #9907, #21164, #31659, #3850, #32620 ) ) ;
#19707=FACE_OUTER_BOUND ( 'NONE', #3995, .T. ) ;
#19724=VECTOR ( 'NONE', #10226, 1000.000000000000114 ) ;
#19735=CARTESIAN_POINT ( 'NONE',  ( -72.05441616160760532, 219.4495263357960368, -2.499999999999991118 ) ) ;
#19764=CARTESIAN_POINT ( 'NONE',  ( -38.47274018782781013, 246.3803829651731121, -0.4999999999999995559 ) ) ;
#19808=VERTEX_POINT ( 'NONE', #15023 ) ;
#19849=CARTESIAN_POINT ( 'NONE',  ( -69.83334449017395684, 223.2245623293732706, -7.500000000000000000 ) ) ;
#19866=ORIENTED_EDGE ( 'NONE', *, *, #25829, .T. ) ;
#19911=EDGE_CURVE ( 'NONE', #4550, #13097, #3645, .T. ) ;
#19913=EDGE_CURVE ( 'NONE', #3827, #15181, #27334, .T. ) ;
#19964=ORIENTED_EDGE ( 'NONE', *, *, #19026, .T. ) ;
#19995=VECTOR ( 'NONE', #9897, 1000.000000000000114 ) ;
#20023=DIRECTION ( 'NONE',  ( 0.000000000000000000, 0.000000000000000000, -1.000000000000000000 ) ) ;
#20025=EDGE_CURVE ( 'NONE', #25851, #28581, #3831, .T. ) ;
#20040=EDGE_CURVE ( 'NONE', #4550, #10335, #24676, .T. ) ;
#20050=AXIS2_PLACEMENT_3D ( 'NONE', #37360, #29209, #14824 ) ;
#20070=LINE ( 'NONE', #5456, #17087 ) ;
#20078=EDGE_CURVE ( 'NONE', #12845, #17150, #796, .T. ) ;
#20103=CARTESIAN_POINT ( 'NONE',  ( 0.000000000000000000, 0.000000000000000000, -5.000000000000000000 ) ) ;
#20137=DIRECTION ( 'NONE',  ( -1.000000000000000000, 0.000000000000000000, 0.000000000000000000 ) ) ;
#20159=ADVANCED_FACE ( 'NONE', ( #27891, #11202 ), #4393, .F. ) ;
#20205=CARTESIAN_POINT ( 'NONE',  ( -51.40635080957665792, 236.9611623878118394, 0.4999999999999997780 ) ) ;
#20232=DIRECTION ( 'NONE',  ( 0.000000000000000000, 0.000000000000000000, -1.000000000000000000 ) ) ;
#20288=DIRECTION ( 'NONE',  ( 0.000000000000000000, 0.000000000000000000, -1.000000000000000000 ) ) ;
#20322=EDGE_CURVE ( 'NONE', #6180, #19808, #5503, .T. ) ;
#20351=FACE_BOUND ( 'NONE', #15899, .T. ) ;
#20377=CARTESIAN_POINT ( 'NONE',  ( -70.65404437008253069, 216.5466800865261234, 7.499999999999999112 ) ) ;
#20439=ADVANCED_FACE ( 'NONE', ( #14807 ), #34886, .T. ) ;
#20476=DIRECTION ( 'NONE',  ( -0.000000000000000000, -0.000000000000000000, 1.000000000000000000 ) ) ;
#20587=VECTOR ( 'NONE', #1550, 1000.000000000000000 ) ;
#20607=DIRECTION ( 'NONE',  ( -0.8083506638593009885, -0.5887012860850802110, 0.000000000000000000 ) ) ;
#20648=ORIENTED_EDGE ( 'NONE', *, *, #5426, .F. ) ;
#20666=AXIS2_PLACEMENT_3D ( 'NONE', #18390, #3967, #9289 ) ;
#20669=CARTESIAN_POINT ( 'NONE',  ( -80.98946968704737515, 222.6276076386831733, 7.500000000000000000 ) ) ;
#20686=ORIENTED_EDGE ( 'NONE', *, *, #1589, .F. ) ;
#20689=AXIS2_PLACEMENT_3D ( 'NONE', #36560, #21298, #10601 ) ;
#20710=VECTOR ( 'NONE', #2246, 1000.000000000000000 ) ;
#20720=CARTESIAN_POINT ( 'NONE',  ( -50.22894823740646331, 235.3444610600932094, -7.500000000000000000 ) ) ;
#20728=EDGE_CURVE ( 'NONE', #14336, #21814, #23693, .T. ) ;
#20738=ORIENTED_EDGE ( 'NONE', *, *, #20933, .F. ) ;
#20740=CARTESIAN_POINT ( 'NONE',  ( -82.45892874490161262, 210.6708926576488921, -5.000000000000000000 ) ) ;
#20785=ORIENTED_EDGE ( 'NONE', *, *, #9857, .T. ) ;
#20793=MANIFOLD_SOLID_BREP ( 'Fillet1', #27737 ) ;
#20837=ORIENTED_EDGE ( 'NONE', *, *, #6712, .T. ) ;
#20892=DIRECTION ( 'NONE',  ( -1.000000000000000000, 0.000000000000000000, 1.636531581110199847E-16 ) ) ;
#20916=LINE ( 'NONE', #20720, #28542 ) ;
#20933=EDGE_CURVE ( 'NONE', #33922, #16460, #11155, .T. ) ;
#20971=FACE_OUTER_BOUND ( 'NONE', #24206, .T. ) ;
#20982=DIRECTION ( 'NONE',  ( -0.000000000000000000, -0.000000000000000000, 1.000000000000000000 ) ) ;
#20996=DIRECTION ( 'NONE',  ( 1.000000000000000000, 0.000000000000000000, 0.000000000000000000 ) ) ;
#21011=CARTESIAN_POINT ( 'NONE',  ( -77.00000000000002842, 210.0000000000000000, 5.000000000000000000 ) ) ;
#21021=PRODUCT_DEFINITION_CONTEXT ( 'detailed design', #21182, 'design' ) ;
#21042=CARTESIAN_POINT ( 'NONE',  ( -81.72704584564827712, 216.6260876520869658, 5.000000000000000000 ) ) ;
#21077=ADVANCED_FACE ( 'NONE', ( #19707 ), #25369, .F. ) ;
#21126=DIRECTION ( 'NONE',  ( 1.000000000000000000, 0.000000000000000000, 0.000000000000000000 ) ) ;
#21164=ORIENTED_EDGE ( 'NONE', *, *, #9364, .T. ) ;
#21182=APPLICATION_CONTEXT ( 'automotive_design' ) ;
#21203=CARTESIAN_POINT ( 'NONE',  ( 0.000000000000000000, 0.000000000000000000, 5.000000000000000000 ) ) ;
#21248=EDGE_LOOP ( 'NONE', ( #2157, #12182 ) ) ;
#21298=DIRECTION ( 'NONE',  ( -0.000000000000000000, -0.000000000000000000, 1.000000000000000000 ) ) ;
#21330=CARTESIAN_POINT ( 'NONE',  ( -77.00000000000002842, 210.0000000000000000, 5.000000000000000888 ) ) ;
#21364=DIRECTION ( 'NONE',  ( -0.000000000000000000, -0.000000000000000000, 1.000000000000000000 ) ) ;
#21377=CIRCLE ( 'NONE', #758, 9.999999999999994671 ) ;
#21389=DIRECTION ( 'NONE',  ( -0.1219804832088933616, -0.9925324990730152175, 0.000000000000000000 ) ) ;
#21438=PLANE ( 'NONE',  #33039 ) ;
#21454=ORIENTED_EDGE ( 'NONE', *, *, #12556, .T. ) ;
#21462=DIRECTION ( 'NONE',  ( -1.558072081575740353E-16, -1.134704379232807653E-16, -1.000000000000000000 ) ) ;
#21478=UNCERTAINTY_MEASURE_WITH_UNIT (LENGTH_MEASURE( 1.000000000000000082E-05 ), #33793, 'distance_accuracy_value', 'NONE');
#21479=ORIENTED_EDGE ( 'NONE', *, *, #33078, .T. ) ;
#21495=CARTESIAN_POINT ( 'NONE',  ( -56.70466238434234185, 244.2363183625454894, 7.500000000000000000 ) ) ;
#21562=VERTEX_POINT ( 'NONE', #13487 ) ;
#21576=DIRECTION ( 'NONE',  ( -0.9925324990730152175, 0.1219804832088933616, 0.000000000000000000 ) ) ;
#21620=DIRECTION ( 'NONE',  ( -0.000000000000000000, -0.000000000000000000, 1.000000000000000000 ) ) ;
#21745=EDGE_LOOP ( 'NONE', ( #37270, #3331, #34586, #27323 ) ) ;
#21746=LINE ( 'NONE', #7337, #16233 ) ;
#21799=EDGE_CURVE ( 'NONE', #19165, #9189, #3999, .T. ) ;
#21813=ORIENTED_EDGE ( 'NONE', *, *, #34811, .T. ) ;
#21814=VERTEX_POINT ( 'NONE', #29523 ) ;
#21854=ORIENTED_EDGE ( 'NONE', *, *, #20078, .T. ) ;
#21878=EDGE_CURVE ( 'NONE', #25851, #1984, #29905, .T. ) ;
#21905=ORIENTED_EDGE ( 'NONE', *, *, #18128, .F. ) ;
#21934=CARTESIAN_POINT ( 'NONE',  ( 0.000000000000000000, 0.000000000000000000, 3.000000000000000000 ) ) ;
#21973=CIRCLE ( 'NONE', #25599, 2.649999999999992806 ) ;
#22001=ORIENTED_EDGE ( 'NONE', *, *, #8440, .T. ) ;
#22032=( GEOMETRIC_REPRESENTATION_CONTEXT ( 3 ) GLOBAL_UNCERTAINTY_ASSIGNED_CONTEXT ( ( #24495 ) ) GLOBAL_UNIT_ASSIGNED_CONTEXT ( ( #13895, #34347, #8945 ) ) REPRESENTATION_CONTEXT ( 'NONE', 'WORKASPACE' ) );
#22054=( NAMED_UNIT ( * ) SI_UNIT ( $, .STERADIAN. ) SOLID_ANGLE_UNIT ( ) );
#22095=ORIENTED_EDGE ( 'NONE', *, *, #26724, .F. ) ;
#22297=VECTOR ( 'NONE', #10460, 1000.000000000000114 ) ;
#22347=EDGE_CURVE ( 'NONE', #13899, #26761, #23376, .T. ) ;
#22363=ADVANCED_FACE ( 'NONE', ( #23944, #32269 ), #29234, .F. ) ;
#22446=CARTESIAN_POINT ( 'NONE',  ( 52.59268362704444399, 124.7349959275252615, 2.500000000000000000 ) ) ;
#22482=EDGE_CURVE ( 'NONE', #10335, #35545, #10796, .T. ) ;
#22507=EDGE_LOOP ( 'NONE', ( #27698, #21905, #34465, #1330 ) ) ;
#22533=CARTESIAN_POINT ( 'NONE',  ( 38.04237167757703020, 114.1383727779938511, 7.500000000000000000 ) ) ;
#22610=ADVANCED_FACE ( 'NONE', ( #16307 ), #33733, .F. ) ;
#22626=VECTOR ( 'NONE', #18871, 1000.000000000000000 ) ;
#22629=EDGE_CURVE ( 'NONE', #21, #4681, #12411, .T. ) ;
#22630=VERTEX_POINT ( 'NONE', #27672 ) ;
#22642=DIRECTION ( 'NONE',  ( 0.1219804832088915436, 0.9925324990730154395, 0.000000000000000000 ) ) ;
#22651=ORIENTED_EDGE ( 'NONE', *, *, #790, .T. ) ;
#22653=VERTEX_POINT ( 'NONE', #4546 ) ;
#22730=PLANE ( 'NONE',  #3138 ) ;
#22734=ORIENTED_EDGE ( 'NONE', *, *, #7408, .F. ) ;
#22768=CARTESIAN_POINT ( 'NONE',  ( -70.80918835584510873, 215.2843023367891249, -7.500000000000000000 ) ) ;
#22859=CARTESIAN_POINT ( 'NONE',  ( -80.75120197997713944, 224.5663476446710831, -7.500000000000000000 ) ) ;
#22866=CARTESIAN_POINT ( 'NONE',  ( -74.35000000000002274, 210.0000000000000000, -5.000000000000001776 ) ) ;
#22881=DIRECTION ( 'NONE',  ( 0.1219804832088915436, 0.9925324990730154395, 0.000000000000000000 ) ) ;
#22885=DIRECTION ( 'NONE',  ( 0.5887012860850814322, -0.8083506638593001004, -3.328006943901143992E-31 ) ) ;
#22891=ADVANCED_FACE ( 'NONE', ( #13046 ), #30291, .F. ) ;
#22943=ADVANCED_FACE ( 'NONE', ( #4316 ), #33878, .T. ) ;
#22976=EDGE_LOOP ( 'NONE', ( #8833, #34974 ) ) ;
#23016=EDGE_CURVE ( 'NONE', #15181, #5473, #19313, .T. ) ;
#23030=VECTOR ( 'NONE', #8017, 1000.000000000000114 ) ;
#23041=DIRECTION ( 'NONE',  ( -0.1219804832088935975, -0.9925324990730152175, 0.000000000000000000 ) ) ;
#23069=DIRECTION ( 'NONE',  ( 1.000000000000000000, 0.000000000000000000, 0.000000000000000000 ) ) ;
#23086=ORIENTED_EDGE ( 'NONE', *, *, #20322, .F. ) ;
#23101=ORIENTED_EDGE ( 'NONE', *, *, #19026, .F. ) ;
#23118=EDGE_CURVE ( 'NONE', #3827, #19208, #8291, .T. ) ;
#23134=CARTESIAN_POINT ( 'NONE',  ( -74.35000000000003695, 210.0000000000000000, 5.000000000000000888 ) ) ;
#23189=DIRECTION ( 'NONE',  ( -1.000000000000000000, 0.000000000000000000, 1.558072081575740353E-16 ) ) ;
#23224=ORIENTED_EDGE ( 'NONE', *, *, #8424, .T. ) ;
#23244=MECHANICAL_DESIGN_GEOMETRIC_PRESENTATION_REPRESENTATION('',(#34112),#22032);
#23257=CARTESIAN_POINT ( 'NONE',  ( -47.00000000000000711, 244.5000000000000000, 0.4999999999999995559 ) ) ;
#23268=DIRECTION ( 'NONE',  ( -0.5887012860850800999, 0.8083506638593009885, -0.000000000000000000 ) ) ;
#23312=CARTESIAN_POINT ( 'NONE',  ( -77.00000000000002842, 210.0000000000000000, 5.000000000000000000 ) ) ;
#23376=LINE ( 'NONE', #15033, #12501 ) ;
#23432=ORIENTED_EDGE ( 'NONE', *, *, #3926, .T. ) ;
#23435=CARTESIAN_POINT ( 'NONE',  ( -79.65000000000001990, 210.0000000000000000, 5.000000000000000000 ) ) ;
#23439=CARTESIAN_POINT ( 'NONE',  ( -38.47274018782780303, 246.3803829651731121, 5.000000000000000000 ) ) ;
#23502=VECTOR ( 'NONE', #9444, 1000.000000000000000 ) ;
#23509=ADVANCED_FACE ( 'NONE', ( #375 ), #28033, .F. ) ;
#23524=AXIS2_PLACEMENT_3D ( 'NONE', #15872, #15493, #4295 ) ;
#23549=EDGE_CURVE ( 'NONE', #30233, #25013, #30134, .T. ) ;
#23600=LINE ( 'NONE', #35145, #1826 ) ;
#23608=AXIS2_PLACEMENT_3D ( 'NONE', #30696, #10591, #13823 ) ;
#23631=EDGE_CURVE ( 'NONE', #17495, #12159, #1688, .T. ) ;
#23654=DIRECTION ( 'NONE',  ( -0.5887012860850802110, 0.8083506638593008775, 0.000000000000000000 ) ) ;
#23693=LINE ( 'NONE', #29744, #10918 ) ;
#23708=CARTESIAN_POINT ( 'NONE',  ( 38.04237167757703020, 114.1383727779938511, 2.500000000000000000 ) ) ;
#23719=EDGE_CURVE ( 'NONE', #33922, #22630, #31436, .T. ) ;
#23733=ORIENTED_EDGE ( 'NONE', *, *, #23549, .F. ) ;
#23739=DIRECTION ( 'NONE',  ( -0.000000000000000000, -0.000000000000000000, -1.000000000000000000 ) ) ;
#23764=ORIENTED_EDGE ( 'NONE', *, *, #18128, .T. ) ;
#23849=CARTESIAN_POINT ( 'NONE',  ( -35.67863628793906372, 245.9410842096246199, -2.499999999999999556 ) ) ;
#23905=ORIENTED_EDGE ( 'NONE', *, *, #5262, .F. ) ;
#23944=FACE_OUTER_BOUND ( 'NONE', #27900, .T. ) ;
#23956=VERTEX_POINT ( 'NONE', #23849 ) ;
#24004=LINE ( 'NONE', #32707, #35345 ) ;
#24037=DIRECTION ( 'NONE',  ( -0.8083506638593009885, -0.5887012860850800999, 1.927470528863119049E-16 ) ) ;
#24048=ORIENTED_EDGE ( 'NONE', *, *, #3104, .F. ) ;
#24072=FACE_OUTER_BOUND ( 'NONE', #22507, .T. ) ;
#24073=LINE ( 'NONE', #3598, #18794 ) ;
#24101=VECTOR ( 'NONE', #23041, 1000.000000000000000 ) ;
#24107=VECTOR ( 'NONE', #1885, 1000.000000000000000 ) ;
#24169=PLANE ( 'NONE',  #28099 ) ;
#24174=EDGE_LOOP ( 'NONE', ( #18964, #10513, #21454, #34888 ) ) ;
#24206=EDGE_LOOP ( 'NONE', ( #33008, #5889, #10889, #8366 ) ) ;
#24209=FACE_OUTER_BOUND ( 'NONE', #21745, .T. ) ;
#24221=DIRECTION ( 'NONE',  ( 0.000000000000000000, 0.000000000000000000, -1.000000000000000000 ) ) ;
#24224=DIRECTION ( 'NONE',  ( -0.8083506638593008775, -0.5887012860850803220, 0.000000000000000000 ) ) ;
#24236=EDGE_LOOP ( 'NONE', ( #30826, #14291, #7222, #28501 ) ) ;
#24364=DIRECTION ( 'NONE',  ( -0.000000000000000000, -0.000000000000000000, -1.000000000000000000 ) ) ;
#24384=CARTESIAN_POINT ( 'NONE',  ( -70.80918835584510873, 215.2843023367891249, 7.500000000000000000 ) ) ;
#24444=( LENGTH_UNIT ( ) NAMED_UNIT ( * ) SI_UNIT ( .MILLI., .METRE. ) );
#24454=EDGE_CURVE ( 'NONE', #37366, #4785, #18218, .T. ) ;
#24489=VECTOR ( 'NONE', #25330, 1000.000000000000000 ) ;
#24495=UNCERTAINTY_MEASURE_WITH_UNIT (LENGTH_MEASURE( 1.000000000000000082E-05 ), #13895, 'distance_accuracy_value', 'NONE');
#24586=CARTESIAN_POINT ( 'NONE',  ( 0.000000000000000000, 0.000000000000000000, 7.500000000000000000 ) ) ;
#24601=DIRECTION ( 'NONE',  ( 0.8083506638593001004, 0.5887012860850814322, -0.000000000000000000 ) ) ;
#24608=DIRECTION ( 'NONE',  ( -0.8083506638593009885, -0.5887012860850802110, 0.000000000000000000 ) ) ;
#24640=ADVANCED_FACE ( 'NONE', ( #384, #26536 ), #21438, .T. ) ;
#24673=ORIENTED_EDGE ( 'NONE', *, *, #7888, .T. ) ;
#24676=LINE ( 'NONE', #26764, #18211 ) ;
#24689=DIRECTION ( 'NONE',  ( 0.000000000000000000, 0.000000000000000000, -1.000000000000000000 ) ) ;
#24720=DIRECTION ( 'NONE',  ( -0.9925324990730152175, 0.1219804832088933616, 0.000000000000000000 ) ) ;
#24775=PLANE ( 'NONE',  #12336 ) ;
#24815=CARTESIAN_POINT ( 'NONE',  ( -98.52697526167153796, 63.53212182842481326, 5.000000000000000000 ) ) ;
#24817=ORIENTED_EDGE ( 'NONE', *, *, #19453, .T. ) ;
#24834=FACE_OUTER_BOUND ( 'NONE', #14634, .T. ) ;
#24858=DIRECTION ( 'NONE',  ( -0.000000000000000000, -0.000000000000000000, 1.000000000000000000 ) ) ;
#24869=LINE ( 'NONE', #36417, #22297 ) ;
#24982=EDGE_CURVE ( 'NONE', #25851, #33921, #10284, .T. ) ;
#24992=( NAMED_UNIT ( * ) PLANE_ANGLE_UNIT ( ) SI_UNIT ( $, .RADIAN. ) );
#25013=VERTEX_POINT ( 'NONE', #9734 ) ;
#25033=AXIS2_PLACEMENT_3D ( 'NONE', #31336, #31519, #3079 ) ;
#25047=DIRECTION ( 'NONE',  ( -0.000000000000000000, 0.000000000000000000, 1.000000000000000000 ) ) ;
#25057=ORIENTED_EDGE ( 'NONE', *, *, #33040, .F. ) ;
#25067=CARTESIAN_POINT ( 'NONE',  ( -74.35000000000002274, 210.0000000000000000, -3.000000000000000000 ) ) ;
#25109=EDGE_LOOP ( 'NONE', ( #26362, #4074, #5134, #35595 ) ) ;
#25159=DIRECTION ( 'NONE',  ( -0.9925324990730154395, 0.1219804832088915297, 0.000000000000000000 ) ) ;
#25165=PLANE ( 'NONE',  #33193 ) ;
#25206=ORIENTED_EDGE ( 'NONE', *, *, #17513, .T. ) ;
#25210=EDGE_CURVE ( 'NONE', #21, #113, #301, .T. ) ;
#25213=PLANE ( 'NONE',  #18623 ) ;
#25218=DIRECTION ( 'NONE',  ( -0.000000000000000000, 0.000000000000000000, 1.000000000000000000 ) ) ;
#25322=PLANE ( 'NONE',  #26511 ) ;
#25330=DIRECTION ( 'NONE',  ( -0.9925324990730152175, 0.1219804832088933616, 0.000000000000000000 ) ) ;
#25369=PLANE ( 'NONE',  #10066 ) ;
#25418=VECTOR ( 'NONE', #29990, 1000.000000000000114 ) ;
#25453=EDGE_CURVE ( 'NONE', #4785, #26761, #27395, .T. ) ;
#25459=ORIENTED_EDGE ( 'NONE', *, *, #25453, .F. ) ;
#25472=DIRECTION ( 'NONE',  ( 0.9925324990730152175, -0.1219804832088933616, 0.000000000000000000 ) ) ;
#25513=LINE ( 'NONE', #37066, #24489 ) ;
#25516=CARTESIAN_POINT ( 'NONE',  ( -60.72871937935236986, 215.3268752544371978, -7.500000000000000888 ) ) ;
#25561=ORIENTED_EDGE ( 'NONE', *, *, #20025, .T. ) ;
#25599=AXIS2_PLACEMENT_3D ( 'NONE', #27861, #28049, #1893 ) ;
#25622=EDGE_CURVE ( 'NONE', #4681, #21, #14879, .T. ) ;
#25626=SURFACE_STYLE_FILL_AREA ( #8206 ) ;
#25668=AXIS2_PLACEMENT_3D ( 'NONE', #15269, #4076, #32320 ) ;
#25669=DIRECTION ( 'NONE',  ( 1.000000000000000000, 0.000000000000000000, 0.000000000000000000 ) ) ;
#25676=AXIS2_PLACEMENT_3D ( 'NONE', #33378, #13668, #4750 ) ;
#25746=ORIENTED_EDGE ( 'NONE', *, *, #23719, .T. ) ;
#25755=VECTOR ( 'NONE', #24689, 1000.000000000000000 ) ;
#25829=EDGE_CURVE ( 'NONE', #26637, #3147, #8611, .T. ) ;
#25851=VERTEX_POINT ( 'NONE', #17707 ) ;
#25874=CARTESIAN_POINT ( 'NONE',  ( -49.64999999999999858, 244.5000000000000000, 2.500000000000000000 ) ) ;
#25880=EDGE_CURVE ( 'NONE', #5473, #25013, #18089, .T. ) ;
#25893=LINE ( 'NONE', #37441, #13672 ) ;
#25901=EDGE_LOOP ( 'NONE', ( #30994, #28549, #14064, #27584 ) ) ;
#25905=DIRECTION ( 'NONE',  ( -0.9925324990730154395, 0.1219804832088915297, 0.000000000000000000 ) ) ;
#25954=CIRCLE ( 'NONE', #23524, 2.649999999999992806 ) ;
#25964=PLANE ( 'NONE',  #15551 ) ;
#25974=DIRECTION ( 'NONE',  ( -0.000000000000000000, -0.000000000000000000, 1.000000000000000000 ) ) ;
#25999=PRESENTATION_STYLE_ASSIGNMENT (( #31685 ) ) ;
#26168=VERTEX_POINT ( 'NONE', #17269 ) ;
#26208=CARTESIAN_POINT ( 'NONE',  ( -70.80918835584510873, 215.2843023367891249, 7.500000000000000000 ) ) ;
#26215=ORIENTED_EDGE ( 'NONE', *, *, #26724, .T. ) ;
#26256=CARTESIAN_POINT ( 'NONE',  ( 6.225801843091343102, 50.65819137209577150, -3.000000000000000000 ) ) ;
#26319=EDGE_CURVE ( 'NONE', #23956, #31856, #28940, .T. ) ;
#26326=FACE_OUTER_BOUND ( 'NONE', #5334, .T. ) ;
#26338=VECTOR ( 'NONE', #32603, 1000.000000000000114 ) ;
#26358=LINE ( 'NONE', #6471, #34760 ) ;
#26362=ORIENTED_EDGE ( 'NONE', *, *, #9673, .T. ) ;
#26390=CARTESIAN_POINT ( 'NONE',  ( -79.65000000000001990, 210.0000000000000000, 3.000000000000000000 ) ) ;
#26458=FACE_OUTER_BOUND ( 'NONE', #6833, .T. ) ;
#26465=ADVANCED_FACE ( 'NONE', ( #15866 ), #12821, .F. ) ;
#26511=AXIS2_PLACEMENT_3D ( 'NONE', #4665, #7524, #19099 ) ;
#26536=FACE_OUTER_BOUND ( 'NONE', #33563, .T. ) ;
#26570=EDGE_LOOP ( 'NONE', ( #23733, #35780, #33432, #6834 ) ) ;
#26637=VERTEX_POINT ( 'NONE', #10482 ) ;
#26671=CARTESIAN_POINT ( 'NONE',  ( -56.70466238434235606, 244.2363183625454894, -7.500000000000000000 ) ) ;
#26714=LINE ( 'NONE', #15733, #19512 ) ;
#26718=EDGE_LOOP ( 'NONE', ( #9703, #6843 ) ) ;
#26724=EDGE_CURVE ( 'NONE', #12557, #11818, #31269, .T. ) ;
#26761=VERTEX_POINT ( 'NONE', #36631 ) ;
#26764=CARTESIAN_POINT ( 'NONE',  ( 38.04237167757722915, 114.1383727779940074, 0.5000000000000000000 ) ) ;
#26811=DIRECTION ( 'NONE',  ( -1.000000000000000000, 0.000000000000000000, 1.636531581110199847E-16 ) ) ;
#26847=CIRCLE ( 'NONE', #25033, 9.999999999999994671 ) ;
#26853=EDGE_LOOP ( 'NONE', ( #11618, #30905, #12800, #3046 ) ) ;
#27021=ORIENTED_EDGE ( 'NONE', *, *, #4942, .T. ) ;
#27055=CYLINDRICAL_SURFACE ( 'NONE', #11000, 2.649999999999999467 ) ;
#27074=ORIENTED_EDGE ( 'NONE', *, *, #8314, .F. ) ;
#27149=DIRECTION ( 'NONE',  ( -0.000000000000000000, -0.000000000000000000, -1.000000000000000000 ) ) ;
#27197=CARTESIAN_POINT ( 'NONE',  ( -42.59364919042334208, 252.0388376121882175, 5.000000000000000000 ) ) ;
#27287=VECTOR ( 'NONE', #20288, 1000.000000000000000 ) ;
#27316=VECTOR ( 'NONE', #14230, 1000.000000000000000 ) ;
#27323=ORIENTED_EDGE ( 'NONE', *, *, #36921, .T. ) ;
#27334=LINE ( 'NONE', #1365, #20587 ) ;
#27389=EDGE_LOOP ( 'NONE', ( #33373, #7734, #5612, #1568 ) ) ;
#27395=LINE ( 'NONE', #27956, #13678 ) ;
#27483=LINE ( 'NONE', #5102, #24107 ) ;
#27490=VECTOR ( 'NONE', #9582, 1000.000000000000000 ) ;
#27544=VECTOR ( 'NONE', #30891, 1000.000000000000114 ) ;
#27573=VERTEX_POINT ( 'NONE', #2469 ) ;
#27584=ORIENTED_EDGE ( 'NONE', *, *, #18763, .F. ) ;
#27672=CARTESIAN_POINT ( 'NONE',  ( -51.40635080957662950, 236.9611623878118110, -0.4999999999999978351 ) ) ;
#27698=ORIENTED_EDGE ( 'NONE', *, *, #676, .F. ) ;
#27726=ORIENTED_EDGE ( 'NONE', *, *, #20040, .T. ) ;
#27730=ADVANCED_FACE ( 'NONE', ( #5314, #34124 ), #25964, .T. ) ;
#27737=CLOSED_SHELL ( 'NONE', ( #29378, #9574, #26465, #4055, #22363, #30691, #8890, #33127, #31420, #27730, #36098, #2063, #7335, #3343, #24640, #165, #21077, #15517, #35849, #11878, #16362, #22891, #22610, #14129, #20159, #2225, #17078, #31832, #33336, #22943, #7750, #20439, #12134, #31495, #4367, #23509, #29315 ) ) ;
#27739=DIRECTION ( 'NONE',  ( -0.000000000000000000, 0.000000000000000000, -1.000000000000000000 ) ) ;
#27743=CARTESIAN_POINT ( 'NONE',  ( -81.72704584564829133, 216.6260876520869658, 7.500000000000000000 ) ) ;
#27793=VERTEX_POINT ( 'NONE', #23134 ) ;
#27800=ADVANCED_BREP_SHAPE_REPRESENTATION ( '', ( #20793, #17215 ), #15973 ) ;
#27813=ORIENTED_EDGE ( 'NONE', *, *, #36921, .F. ) ;
#27841=CARTESIAN_POINT ( 'NONE',  ( -89.59418277001438469, 62.43429747954478159, 5.000000000000000000 ) ) ;
#27854=CARTESIAN_POINT ( 'NONE',  ( -77.35272773637332477, 226.7246823105297153, 0.4999999999999995559 ) ) ;
#27861=CARTESIAN_POINT ( 'NONE',  ( -47.00000000000000711, 244.5000000000000000, 0.4999999999999995559 ) ) ;
#27869=AXIS2_PLACEMENT_3D ( 'NONE', #29301, #2967, #20607 ) ;
#27891=FACE_BOUND ( 'NONE', #22976, .T. ) ;
#27900=EDGE_LOOP ( 'NONE', ( #27074, #32702, #9823, #19964, #10238, #23764, #29430, #3848 ) ) ;
#27956=CARTESIAN_POINT ( 'NONE',  ( -70.80918835584510873, 215.2843023367891249, 7.500000000000000000 ) ) ;
#27979=CARTESIAN_POINT ( 'NONE',  ( -79.74198084750223359, 216.3821266856691636, -3.000000000000000000 ) ) ;
#28004=ORIENTED_EDGE ( 'NONE', *, *, #24982, .F. ) ;
#28021=VECTOR ( 'NONE', #3879, 1000.000000000000000 ) ;
#28029=VECTOR ( 'NONE', #24037, 1000.000000000000000 ) ;
#28030=LINE ( 'NONE', #16670, #20710 ) ;
#28033=CYLINDRICAL_SURFACE ( 'NONE', #3950, 10.00000000000000178 ) ;
#28049=DIRECTION ( 'NONE',  ( -0.000000000000000000, 0.000000000000000000, 1.000000000000000000 ) ) ;
#28099=AXIS2_PLACEMENT_3D ( 'NONE', #32877, #18303, #6924 ) ;
#28158=ORIENTED_EDGE ( 'NONE', *, *, #2412, .T. ) ;
#28170=FACE_OUTER_BOUND ( 'NONE', #30800, .T. ) ;
#28178=ORIENTED_EDGE ( 'NONE', *, *, #18405, .T. ) ;
#28195=VECTOR ( 'NONE', #442, 1000.000000000000000 ) ;
#28217=AXIS2_PLACEMENT_3D ( 'NONE', #12086, #35022, #6217 ) ;
#28265=DIRECTION ( 'NONE',  ( 1.000000000000000000, 0.000000000000000000, 0.000000000000000000 ) ) ;
#28285=SURFACE_SIDE_STYLE ('',( #25626 ) ) ;
#28294=PRODUCT ( 'handle', 'handle', '', ( #15295 ) ) ;
#28465=DIRECTION ( 'NONE',  ( 0.000000000000000000, 0.000000000000000000, -1.000000000000000000 ) ) ;
#28471=EDGE_LOOP ( 'NONE', ( #23224, #12901 ) ) ;
#28501=ORIENTED_EDGE ( 'NONE', *, *, #19913, .F. ) ;
#28531=CARTESIAN_POINT ( 'NONE',  ( -55.52725981217218276, 242.6196170348268879, 5.000000000000000000 ) ) ;
#28542=VECTOR ( 'NONE', #29424, 1000.000000000000114 ) ;
#28549=ORIENTED_EDGE ( 'NONE', *, *, #23549, .T. ) ;
#28581=VERTEX_POINT ( 'NONE', #8121 ) ;
#28625=CARTESIAN_POINT ( 'NONE',  ( -49.64999999999999858, 244.5000000000000000, 5.000000000000000000 ) ) ;
#28643=EDGE_LOOP ( 'NONE', ( #12192, #30854, #12743, #20686, #4661, #31176, #2544, #9495 ) ) ;
#28650=CYLINDRICAL_SURFACE ( 'NONE', #10128, 9.999999999999994671 ) ;
#28674=CARTESIAN_POINT ( 'NONE',  ( -82.45892874490161262, 210.6708926576488921, 5.000000000000000000 ) ) ;
#28736=ORIENTED_EDGE ( 'NONE', *, *, #16456, .F. ) ;
#28756=FACE_OUTER_BOUND ( 'NONE', #8021, .T. ) ;
#28885=LINE ( 'NONE', #14865, #11150 ) ;
#28931=PLANE ( 'NONE',  #27869 ) ;
#28940=LINE ( 'NONE', #11695, #17338 ) ;
#28968=VERTEX_POINT ( 'NONE', #24384 ) ;
#29004=ORIENTED_EDGE ( 'NONE', *, *, #9673, .F. ) ;
#29035=LINE ( 'NONE', #8776, #31682 ) ;
#29160=EDGE_CURVE ( 'NONE', #10660, #1475, #1057, .T. ) ;
#29163=EDGE_CURVE ( 'NONE', #9189, #33064, #9787, .T. ) ;
#29164=DIRECTION ( 'NONE',  ( 1.000000000000000000, 0.000000000000000000, 0.000000000000000000 ) ) ;
#29209=DIRECTION ( 'NONE',  ( 0.000000000000000000, 0.000000000000000000, -1.000000000000000000 ) ) ;
#29228=VECTOR ( 'NONE', #13580, 1000.000000000000000 ) ;
#29234=PLANE ( 'NONE',  #14314 ) ;
#29291=AXIS2_PLACEMENT_3D ( 'NONE', #14095, #13914, #1782 ) ;
#29301=CARTESIAN_POINT ( 'NONE',  ( -77.35272773637332477, 226.7246823105297153, 5.000000000000000000 ) ) ;
#29315=ADVANCED_FACE ( 'NONE', ( #31684 ), #28650, .T. ) ;
#29370=VECTOR ( 'NONE', #22881, 1000.000000000000000 ) ;
#29378=ADVANCED_FACE ( 'NONE', ( #13709 ), #31318, .F. ) ;
#29424=DIRECTION ( 'NONE',  ( -0.8083506638593008775, -0.5887012860850803220, 0.000000000000000000 ) ) ;
#29429=DIRECTION ( 'NONE',  ( -0.9925324990730154395, 0.1219804832088915297, 0.000000000000000000 ) ) ;
#29430=ORIENTED_EDGE ( 'NONE', *, *, #33045, .T. ) ;
#29467=CARTESIAN_POINT ( 'NONE',  ( -70.65404437008254490, 216.5466800865261234, -7.500000000000000000 ) ) ;
#29506=ORIENTED_EDGE ( 'NONE', *, *, #31547, .F. ) ;
#29522=CARTESIAN_POINT ( 'NONE',  ( -42.15435043487492095, 254.8329415120769283, -2.500000000000000000 ) ) ;
#29523=CARTESIAN_POINT ( 'NONE',  ( -35.67863628793906372, 245.9410842096246199, 2.500000000000000000 ) ) ;
#29567=EDGE_LOOP ( 'NONE', ( #25459, #14112, #1664, #29506 ) ) ;
#29654=DIRECTION ( 'NONE',  ( -0.8083506638593008775, -0.5887012860850803220, 0.000000000000000000 ) ) ;
#29689=AXIS2_PLACEMENT_3D ( 'NONE', #7811, #25047, #28265 ) ;
#29703=DIRECTION ( 'NONE',  ( 1.000000000000000000, 0.000000000000000000, 0.000000000000000000 ) ) ;
#29744=CARTESIAN_POINT ( 'NONE',  ( -72.05441616160760532, 219.4495263357960368, 2.500000000000000000 ) ) ;
#29745=CYLINDRICAL_SURFACE ( 'NONE', #17043, 2.649999999999999467 ) ;
#29763=ORIENTED_EDGE ( 'NONE', *, *, #20728, .F. ) ;
#29773=VECTOR ( 'NONE', #2574, 1000.000000000000000 ) ;
#29882=CARTESIAN_POINT ( 'NONE',  ( -77.00000000000002842, 210.0000000000000000, 5.000000000000000000 ) ) ;
#29905=LINE ( 'NONE', #12659, #11283 ) ;
#29990=DIRECTION ( 'NONE',  ( 0.5887012860850814322, -0.8083506638592999893, 0.000000000000000000 ) ) ;
#30076=LINE ( 'NONE', #15683, #29228 ) ;
#30128=CARTESIAN_POINT ( 'NONE',  ( -77.00000000000002842, 210.0000000000000000, 5.000000000000000000 ) ) ;
#30134=LINE ( 'NONE', #4165, #19724 ) ;
#30156=ORIENTED_EDGE ( 'NONE', *, *, #20025, .F. ) ;
#30219=DIRECTION ( 'NONE',  ( 1.000000000000000000, 0.000000000000000000, 0.000000000000000000 ) ) ;
#30233=VERTEX_POINT ( 'NONE', #19230 ) ;
#30291=PLANE ( 'NONE',  #916 ) ;
#30381=VECTOR ( 'NONE', #23654, 1000.000000000000114 ) ;
#30462=DIRECTION ( 'NONE',  ( -0.000000000000000000, -0.000000000000000000, 1.000000000000000000 ) ) ;
#30464=CARTESIAN_POINT ( 'NONE',  ( -81.72704584564829133, 216.6260876520869658, -7.500000000000000000 ) ) ;
#30530=VECTOR ( 'NONE', #24364, 1000.000000000000000 ) ;
#30531=CARTESIAN_POINT ( 'NONE',  ( -56.70466238434234185, 244.2363183625454894, -2.499999999999996447 ) ) ;
#30639=VECTOR ( 'NONE', #2988, 1000.000000000000114 ) ;
#30660=DIRECTION ( 'NONE',  ( -0.000000000000000000, -0.000000000000000000, 1.000000000000000000 ) ) ;
#30691=ADVANCED_FACE ( 'NONE', ( #24834 ), #25213, .T. ) ;
#30696=CARTESIAN_POINT ( 'NONE',  ( -77.00000000000002842, 210.0000000000000000, 3.000000000000000000 ) ) ;
#30724=EDGE_LOOP ( 'NONE', ( #35090, #6179 ) ) ;
#30740=EDGE_CURVE ( 'NONE', #23956, #10660, #16879, .T. ) ;
#30741=DIRECTION ( 'NONE',  ( 0.000000000000000000, 0.000000000000000000, -1.000000000000000000 ) ) ;
#30800=EDGE_LOOP ( 'NONE', ( #3707, #12576, #6342, #4736, #36094, #20785, #1788, #30156 ) ) ;
#30802=VERTEX_POINT ( 'NONE', #10596 ) ;
#30826=ORIENTED_EDGE ( 'NONE', *, *, #23118, .T. ) ;
#30851=CARTESIAN_POINT ( 'NONE',  ( -100.7560012262353411, 61.79101779669657191, 5.000000000000000000 ) ) ;
#30854=ORIENTED_EDGE ( 'NONE', *, *, #3349, .T. ) ;
#30855=ORIENTED_EDGE ( 'NONE', *, *, #21878, .F. ) ;
#30891=DIRECTION ( 'NONE',  ( 0.8083506638593009885, 0.5887012860850802110, 0.000000000000000000 ) ) ;
#30905=ORIENTED_EDGE ( 'NONE', *, *, #22347, .F. ) ;
#30994=ORIENTED_EDGE ( 'NONE', *, *, #5518, .F. ) ;
#31026=LINE ( 'NONE', #19849, #1483 ) ;
#31040=CARTESIAN_POINT ( 'NONE',  ( -56.70466238434235606, 244.2363183625454894, 7.500000000000000000 ) ) ;
#31065=CARTESIAN_POINT ( 'NONE',  ( -43.77105176259354380, 253.6555389399068190, 5.000000000000000000 ) ) ;
#31176=ORIENTED_EDGE ( 'NONE', *, *, #23016, .F. ) ;
#31178=EDGE_LOOP ( 'NONE', ( #24817, #21813, #30855, #19154, #3099, #5989, #8233, #31671 ) ) ;
#31197=DIRECTION ( 'NONE',  ( -1.558072081575740353E-16, -1.134704379232807653E-16, -1.000000000000000000 ) ) ;
#31269=CIRCLE ( 'NONE', #11273, 9.999999999999994671 ) ;
#31291=CARTESIAN_POINT ( 'NONE',  ( -51.40635080957662950, 236.9611623878118110, 5.000000000000000000 ) ) ;
#31318=CYLINDRICAL_SURFACE ( 'NONE', #31901, 2.649999999999992806 ) ;
#31336=CARTESIAN_POINT ( 'NONE',  ( -71.06414469631722852, 221.4078028065942476, 7.500000000000000000 ) ) ;
#31365=CIRCLE ( 'NONE', #7785, 2.649999999999985700 ) ;
#31420=ADVANCED_FACE ( 'NONE', ( #6982, #9626 ), #36325, .F. ) ;
#31436=LINE ( 'NONE', #17040, #13650 ) ;
#31481=CARTESIAN_POINT ( 'NONE',  ( -56.70466238434234185, 244.2363183625454894, -2.499999999999996447 ) ) ;
#31495=ADVANCED_FACE ( 'NONE', ( #1652 ), #24775, .T. ) ;
#31519=DIRECTION ( 'NONE',  ( 0.000000000000000000, -0.000000000000000000, 1.000000000000000000 ) ) ;
#31547=EDGE_CURVE ( 'NONE', #26761, #12005, #6592, .T. ) ;
#31590=AXIS2_PLACEMENT_3D ( 'NONE', #24586, #16068, #13780 ) ;
#31659=ORIENTED_EDGE ( 'NONE', *, *, #31837, .T. ) ;
#31665=CARTESIAN_POINT ( 'NONE',  ( -49.64999999999999858, 244.5000000000000000, -2.499999999999997335 ) ) ;
#31671=ORIENTED_EDGE ( 'NONE', *, *, #16982, .T. ) ;
#31682=VECTOR ( 'NONE', #5920, 1000.000000000000000 ) ;
#31684=FACE_OUTER_BOUND ( 'NONE', #32050, .T. ) ;
#31685=SURFACE_STYLE_USAGE ( .BOTH. , #28285 ) ;
#31708=FACE_OUTER_BOUND ( 'NONE', #37353, .T. ) ;
#31715=DIRECTION ( 'NONE',  ( -0.1219804832088933616, -0.9925324990730152175, 0.000000000000000000 ) ) ;
#31747=LINE ( 'NONE', #11103, #9562 ) ;
#31832=ADVANCED_FACE ( 'NONE', ( #13967 ), #33680, .F. ) ;
#31837=EDGE_CURVE ( 'NONE', #3147, #4722, #5063, .T. ) ;
#31848=AXIS2_PLACEMENT_3D ( 'NONE', #29882, #6385, #20996 ) ;
#31856=VERTEX_POINT ( 'NONE', #10742 ) ;
#31901=AXIS2_PLACEMENT_3D ( 'NONE', #5346, #16924, #2501 ) ;
#31938=CARTESIAN_POINT ( 'NONE',  ( 38.04237167757703020, 114.1383727779938511, -2.499999999999996447 ) ) ;
#31983=AXIS2_PLACEMENT_3D ( 'NONE', #32683, #1594, #26811 ) ;
#32050=EDGE_LOOP ( 'NONE', ( #20648, #35751, #22095, #19264 ) ) ;
#32059=FACE_BOUND ( 'NONE', #28471, .T. ) ;
#32163=EDGE_CURVE ( 'NONE', #6034, #14163, #18498, .T. ) ;
#32269=FACE_BOUND ( 'NONE', #26853, .T. ) ;
#32270=ORIENTED_EDGE ( 'NONE', *, *, #31547, .T. ) ;
#32281=ORIENTED_EDGE ( 'NONE', *, *, #26319, .T. ) ;
#32320=DIRECTION ( 'NONE',  ( -1.000000000000000000, 0.000000000000000000, 1.558072081575740353E-16 ) ) ;
#32366=ORIENTED_EDGE ( 'NONE', *, *, #790, .F. ) ;
#32459=DIRECTION ( 'NONE',  ( 0.1219804832088915297, 0.9925324990730154395, 0.000000000000000000 ) ) ;
#32553=AXIS2_PLACEMENT_3D ( 'NONE', #8446, #31197, #2932 ) ;
#32603=DIRECTION ( 'NONE',  ( 0.1219804832088915297, 0.9925324990730154395, 0.000000000000000000 ) ) ;
#32620=ORIENTED_EDGE ( 'NONE', *, *, #18763, .T. ) ;
#32683=CARTESIAN_POINT ( 'NONE',  ( -47.00000000000000711, 244.5000000000000000, -0.4999999999999978351 ) ) ;
#32702=ORIENTED_EDGE ( 'NONE', *, *, #33040, .T. ) ;
#32707=CARTESIAN_POINT ( 'NONE',  ( -79.74198084750223359, 216.3821266856691636, 5.000000000000000000 ) ) ;
#32722=VECTOR ( 'NONE', #25974, 1000.000000000000000 ) ;
#32744=VERTEX_POINT ( 'NONE', #7866 ) ;
#32877=CARTESIAN_POINT ( 'NONE',  ( -78.53013030854349097, 228.3413836382483169, 5.000000000000000000 ) ) ;
#32884=LINE ( 'NONE', #12795, #30530 ) ;
#32903=CARTESIAN_POINT ( 'NONE',  ( -79.65000000000001990, 210.0000000000000000, 5.000000000000000000 ) ) ;
#32971=DIRECTION ( 'NONE',  ( 1.000000000000000000, 0.000000000000000000, 0.000000000000000000 ) ) ;
#33008=ORIENTED_EDGE ( 'NONE', *, *, #30740, .T. ) ;
#33039=AXIS2_PLACEMENT_3D ( 'NONE', #23708, #9859, #12702 ) ;
#33040=EDGE_CURVE ( 'NONE', #4722, #32744, #17712, .T. ) ;
#33045=EDGE_CURVE ( 'NONE', #21562, #30233, #28885, .T. ) ;
#33064=VERTEX_POINT ( 'NONE', #1716 ) ;
#33071=FACE_OUTER_BOUND ( 'NONE', #31178, .T. ) ;
#33078=EDGE_CURVE ( 'NONE', #1071, #14163, #17219, .T. ) ;
#33127=ADVANCED_FACE ( 'NONE', ( #36769 ), #19178, .F. ) ;
#33193=AXIS2_PLACEMENT_3D ( 'NONE', #10946, #36342, #24608 ) ;
#33249=ORIENTED_EDGE ( 'NONE', *, *, #8678, .F. ) ;
#33265=DIRECTION ( 'NONE',  ( -0.000000000000000000, 0.000000000000000000, -1.000000000000000000 ) ) ;
#33301=VECTOR ( 'NONE', #8362, 1000.000000000000000 ) ;
#33336=ADVANCED_FACE ( 'NONE', ( #13350 ), #1965, .F. ) ;
#33373=ORIENTED_EDGE ( 'NONE', *, *, #29160, .T. ) ;
#33378=CARTESIAN_POINT ( 'NONE',  ( -72.05441616160760532, 219.4495263357960368, 5.000000000000000000 ) ) ;
#33419=VECTOR ( 'NONE', #12316, 1000.000000000000000 ) ;
#33432=ORIENTED_EDGE ( 'NONE', *, *, #676, .T. ) ;
#33443=EDGE_LOOP ( 'NONE', ( #23086, #14236, #10384, #19584 ) ) ;
#33524=AXIS2_PLACEMENT_3D ( 'NONE', #25516, #10928, #34050 ) ;
#33563=EDGE_LOOP ( 'NONE', ( #12718, #36380, #4825, #34320 ) ) ;
#33680=CYLINDRICAL_SURFACE ( 'NONE', #8714, 2.649999999999992806 ) ;
#33733=PLANE ( 'NONE',  #11193 ) ;
#33793=( LENGTH_UNIT ( ) NAMED_UNIT ( * ) SI_UNIT ( .MILLI., .METRE. ) );
#33878=PLANE ( 'NONE',  #37243 ) ;
#33920=STYLED_ITEM('',(#37535),#20793);
#33921=VERTEX_POINT ( 'NONE', #16347 ) ;
#33922=VERTEX_POINT ( 'NONE', #19764 ) ;
#33967=VECTOR ( 'NONE', #23739, 1000.000000000000000 ) ;
#33993=DIRECTION ( 'NONE',  ( -0.5887012860850800999, 0.8083506638593009885, -0.000000000000000000 ) ) ;
#34014=CARTESIAN_POINT ( 'NONE',  ( -66.61573224020317241, 223.4103818930302054, -7.499999999999997335 ) ) ;
#34050=DIRECTION ( 'NONE',  ( -1.000000000000000000, 2.775557561562892929E-15, 0.000000000000000000 ) ) ;
#34063=ORIENTED_EDGE ( 'NONE', *, *, #10394, .F. ) ;
#34112=STYLED_ITEM ( 'NONE', ( #25999 ), #27800 ) ;
#34124=FACE_BOUND ( 'NONE', #11079, .T. ) ;
#34162=SHAPE_REPRESENTATION_RELATIONSHIP ( 'NONE' , 'NONE' ,  #2638, #27800 ) ;
#34182=CARTESIAN_POINT ( 'NONE',  ( -100.7560012262353411, 61.79101779669657191, -5.000000000000000000 ) ) ;
#34192=EDGE_CURVE ( 'NONE', #12159, #12005, #24869, .T. ) ;
#34221=LINE ( 'NONE', #22859, #24101 ) ;
#34320=ORIENTED_EDGE ( 'NONE', *, *, #4942, .F. ) ;
#34347=( NAMED_UNIT ( * ) PLANE_ANGLE_UNIT ( ) SI_UNIT ( $, .RADIAN. ) );
#34465=ORIENTED_EDGE ( 'NONE', *, *, #19913, .T. ) ;
#34515=DIRECTION ( 'NONE',  ( -1.000000000000000000, 0.000000000000000000, 0.000000000000000000 ) ) ;
#34586=ORIENTED_EDGE ( 'NONE', *, *, #8705, .T. ) ;
#34605=DIRECTION ( 'NONE',  ( 0.8083506638593009885, 0.5887012860850800999, 0.000000000000000000 ) ) ;
#34640=LINE ( 'NONE', #26671, #9334 ) ;
#34663=AXIS2_PLACEMENT_3D ( 'NONE', #16222, #4643, #15661 ) ;
#34736=CARTESIAN_POINT ( 'NONE',  ( 52.59268362704444399, 124.7349959275252615, -0.5000000000000000000 ) ) ;
#34760=VECTOR ( 'NONE', #35260, 1000.000000000000114 ) ;
#34791=DIRECTION ( 'NONE',  ( -1.558072081575740353E-16, -1.134704379232807653E-16, -1.000000000000000000 ) ) ;
#34811=EDGE_CURVE ( 'NONE', #11818, #1984, #27483, .T. ) ;
#34843=AXIS2_PLACEMENT_3D ( 'NONE', #11082, #16598, #25669 ) ;
#34886=PLANE ( 'NONE',  #16986 ) ;
#34888=ORIENTED_EDGE ( 'NONE', *, *, #1759, .F. ) ;
#34925=DIRECTION ( 'NONE',  ( -0.1219804832088915297, -0.9925324990730154395, 0.000000000000000000 ) ) ;
#34966=LINE ( 'NONE', #31938, #29773 ) ;
#34974=ORIENTED_EDGE ( 'NONE', *, *, #9936, .T. ) ;
#34988=DIRECTION ( 'NONE',  ( 0.000000000000000000, 0.000000000000000000, 1.000000000000000000 ) ) ;
#34994=AXIS2_PLACEMENT_3D ( 'NONE', #23257, #118, #23069 ) ;
#35007=ORIENTED_EDGE ( 'NONE', *, *, #25622, .F. ) ;
#35022=DIRECTION ( 'NONE',  ( 0.000000000000000000, 0.000000000000000000, -1.000000000000000000 ) ) ;
#35090=ORIENTED_EDGE ( 'NONE', *, *, #18405, .F. ) ;
#35121=ORIENTED_EDGE ( 'NONE', *, *, #6712, .F. ) ;
#35145=CARTESIAN_POINT ( 'NONE',  ( -56.70466238434235606, 244.2363183625454894, -7.500000000000000000 ) ) ;
#35167=ORIENTED_EDGE ( 'NONE', *, *, #18419, .F. ) ;
#35215=ORIENTED_EDGE ( 'NONE', *, *, #16456, .T. ) ;
#35260=DIRECTION ( 'NONE',  ( 0.1219804832088915297, 0.9925324990730154395, 0.000000000000000000 ) ) ;
#35331=CARTESIAN_POINT ( 'NONE',  ( 38.04237167757703020, 114.1383727779938511, 2.500000000000000000 ) ) ;
#35345=VECTOR ( 'NONE', #34988, 1000.000000000000000 ) ;
#35396=CARTESIAN_POINT ( 'NONE',  ( -69.83334449017395684, 223.2245623293732706, 7.500000000000000000 ) ) ;
#35427=DIRECTION ( 'NONE',  ( 0.8083506638593009885, 0.5887012860850802110, 0.000000000000000000 ) ) ;
#35466=ORIENTED_EDGE ( 'NONE', *, *, #22629, .F. ) ;
#35496=EDGE_CURVE ( 'NONE', #32744, #28968, #36096, .T. ) ;
#35525=VECTOR ( 'NONE', #35741, 1000.000000000000000 ) ;
#35537=FACE_BOUND ( 'NONE', #7819, .T. ) ;
#35545=VERTEX_POINT ( 'NONE', #10326 ) ;
#35595=ORIENTED_EDGE ( 'NONE', *, *, #19147, .T. ) ;
#35655=CARTESIAN_POINT ( 'NONE',  ( -89.59418277001438469, 62.43429747954478159, -3.000000000000000000 ) ) ;
#35741=DIRECTION ( 'NONE',  ( 0.000000000000000000, 0.000000000000000000, -1.000000000000000000 ) ) ;
#35747=MECHANICAL_DESIGN_GEOMETRIC_PRESENTATION_REPRESENTATION('',(#33920),#14545);
#35751=ORIENTED_EDGE ( 'NONE', *, *, #34811, .F. ) ;
#35755=DIRECTION ( 'NONE',  ( 0.000000000000000000, 0.000000000000000000, -1.000000000000000000 ) ) ;
#35780=ORIENTED_EDGE ( 'NONE', *, *, #33045, .F. ) ;
#35797=VECTOR ( 'NONE', #11857, 1000.000000000000000 ) ;
#35849=ADVANCED_FACE ( 'NONE', ( #7926 ), #25165, .T. ) ;
#35906=EDGE_LOOP ( 'NONE', ( #12856, #19866, #2564, #36848, #11622, #10540, #29763, #7436 ) ) ;
#35934=SHAPE_DEFINITION_REPRESENTATION ( #14397, #2638 ) ;
#36012=ORIENTED_EDGE ( 'NONE', *, *, #7408, .T. ) ;
#36051=EDGE_CURVE ( 'NONE', #6034, #30802, #13831, .T. ) ;
#36094=ORIENTED_EDGE ( 'NONE', *, *, #35496, .F. ) ;
#36096=LINE ( 'NONE', #35396, #23502 ) ;
#36098=ADVANCED_FACE ( 'NONE', ( #37272 ), #37086, .T. ) ;
#36222=DIRECTION ( 'NONE',  ( 1.000000000000000000, 0.000000000000000000, 0.000000000000000000 ) ) ;
#36226=AXIS2_PLACEMENT_3D ( 'NONE', #21934, #35755, #9799 ) ;
#36314=CIRCLE ( 'NONE', #8488, 2.649999999999985700 ) ;
#36317=EDGE_CURVE ( 'NONE', #12005, #26168, #24004, .T. ) ;
#36325=PLANE ( 'NONE',  #14160 ) ;
#36342=DIRECTION ( 'NONE',  ( -0.5887012860850802110, 0.8083506638593009885, 0.000000000000000000 ) ) ;
#36380=ORIENTED_EDGE ( 'NONE', *, *, #5262, .T. ) ;
#36390=EDGE_LOOP ( 'NONE', ( #11667, #25057, #15870, #3423 ) ) ;
#36417=CARTESIAN_POINT ( 'NONE',  ( -104.7527771047627994, 12.87393045632884636, -3.000000000000000000 ) ) ;
#36466=CARTESIAN_POINT ( 'NONE',  ( -60.72871937935236986, 215.3268752544371978, 7.500000000000000000 ) ) ;
#36549=( NAMED_UNIT ( * ) SI_UNIT ( $, .STERADIAN. ) SOLID_ANGLE_UNIT ( ) );
#36560=CARTESIAN_POINT ( 'NONE',  ( -47.00000000000000711, 244.5000000000000000, 5.000000000000000000 ) ) ;
#36631=CARTESIAN_POINT ( 'NONE',  ( -70.80918835584510873, 215.2843023367891249, -2.999999999999999112 ) ) ;
#36769=FACE_OUTER_BOUND ( 'NONE', #35906, .T. ) ;
#36848=ORIENTED_EDGE ( 'NONE', *, *, #29160, .F. ) ;
#36886=EDGE_LOOP ( 'NONE', ( #9689, #32270, #2857, #29004 ) ) ;
#36921=EDGE_CURVE ( 'NONE', #17495, #26168, #26358, .T. ) ;
#36939=ORIENTED_EDGE ( 'NONE', *, *, #4577, .F. ) ;
#36962=VECTOR ( 'NONE', #22885, 999.9999999999998863 ) ;
#37022=LINE ( 'NONE', #28674, #17575 ) ;
#37031=ORIENTED_EDGE ( 'NONE', *, *, #34192, .T. ) ;
#37059=FACE_OUTER_BOUND ( 'NONE', #25901, .T. ) ;
#37064=LINE ( 'NONE', #28531, #6146 ) ;
#37066=CARTESIAN_POINT ( 'NONE',  ( -70.80918835584510873, 215.2843023367891249, 7.500000000000000000 ) ) ;
#37086=PLANE ( 'NONE',  #3805 ) ;
#37243=AXIS2_PLACEMENT_3D ( 'NONE', #31040, #24601, #1846 ) ;
#37260=CARTESIAN_POINT ( 'NONE',  ( -47.00000000000000711, 244.5000000000000000, -2.499999999999997780 ) ) ;
#37267=EDGE_CURVE ( 'NONE', #27573, #1475, #34640, .T. ) ;
#37270=ORIENTED_EDGE ( 'NONE', *, *, #2926, .F. ) ;
#37272=FACE_OUTER_BOUND ( 'NONE', #28643, .T. ) ;
#37353=EDGE_LOOP ( 'NONE', ( #1274, #25206, #10492, #19607 ) ) ;
#37360=CARTESIAN_POINT ( 'NONE',  ( 0.000000000000000000, 0.000000000000000000, -3.000000000000000000 ) ) ;
#37366=VERTEX_POINT ( 'NONE', #12081 ) ;
#37408=CARTESIAN_POINT ( 'NONE',  ( -47.00000000000000711, 244.5000000000000000, 2.500000000000000000 ) ) ;
#37441=CARTESIAN_POINT ( 'NONE',  ( -56.70466238434234185, 244.2363183625454894, 2.500000000000000000 ) ) ;
#37529=COLOUR_RGB('Sky Blue',0.24,0.69,0.87);
#37530=FILL_AREA_STYLE_COLOUR('',#37529);
#37531=FILL_AREA_STYLE('',(#37530));
#37532=SURFACE_STYLE_FILL_AREA(#37531);
#37533=SURFACE_SIDE_STYLE('',(#37532));
#37534=SURFACE_STYLE_USAGE(.BOTH.,#37533);
#37535=PRESENTATION_STYLE_ASSIGNMENT((#37534));
ENDSEC;
END-ISO-10303-21;
